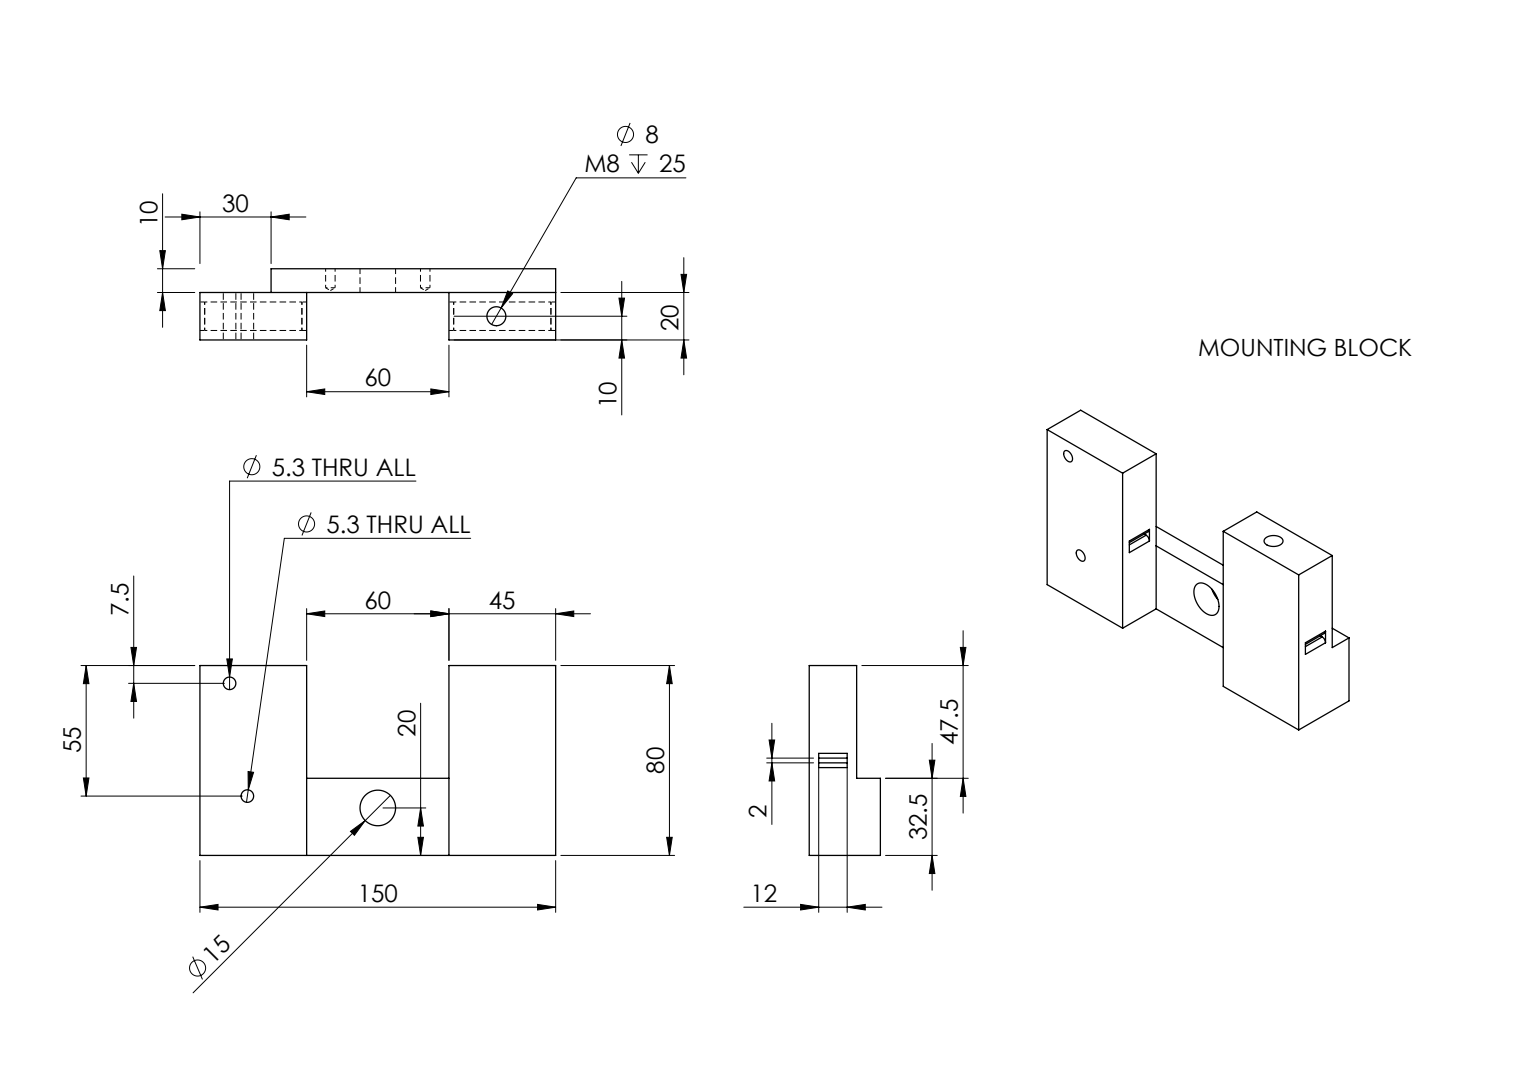
ISO-10303-21;
HEADER;
FILE_DESCRIPTION (('STEP AP214'),
    '1' );
FILE_NAME ('Mounting block.step',
    '2026-10-31T03:44:21',
    ( '' ),
    ( '' ),
    'SwSTEP 2.0',
    'SolidWorks 2026',
    '' );
FILE_SCHEMA (( 'AUTOMOTIVE_DESIGN' ));
ENDSEC;

DATA;
#10=VECTOR ( 'NONE', #15032, 1000.000000000000000 ) ;
#26=CIRCLE ( 'NONE', #5977, 1.999999999999998224 ) ;
#31=DIRECTION ( 'NONE',  ( -0.000000000000000000, 1.000000000000000000, -0.000000000000000000 ) ) ;
#35=DIRECTION ( 'NONE',  ( -1.000000000000000000, 0.000000000000000000, 0.000000000000000000 ) ) ;
#45=ORIENTED_EDGE ( 'NONE', *, *, #3522, .F. ) ;
#50=EDGE_CURVE ( 'NONE', #8587, #13131, #8250, .T. ) ;
#54=VECTOR ( 'NONE', #3678, 1000.000000000000000 ) ;
#66=DIRECTION ( 'NONE',  ( -1.000000000000000000, 0.000000000000000000, 0.000000000000000000 ) ) ;
#98=EDGE_LOOP ( 'NONE', ( #16825, #4410, #16982, #5745 ) ) ;
#99=DIRECTION ( 'NONE',  ( -1.000000000000000000, 0.000000000000000000, -0.000000000000000000 ) ) ;
#101=CARTESIAN_POINT ( 'NONE',  ( -74.99999999999997158, 1.000000000000000000, -5.999999999999998224 ) ) ;
#107=FACE_OUTER_BOUND ( 'NONE', #1049, .T. ) ;
#122=DIRECTION ( 'NONE',  ( -1.000000000000000000, 0.000000000000000000, 0.000000000000000000 ) ) ;
#140=LINE ( 'NONE', #4756, #15155 ) ;
#151=ORIENTED_EDGE ( 'NONE', *, *, #16122, .F. ) ;
#168=EDGE_CURVE ( 'NONE', #12513, #18552, #6292, .T. ) ;
#192=ADVANCED_FACE ( 'NONE', ( #13732 ), #15592, .F. ) ;
#220=DIRECTION ( 'NONE',  ( 0.000000000000000000, 0.000000000000000000, -1.000000000000000000 ) ) ;
#224=ADVANCED_FACE ( 'NONE', ( #6567 ), #9413, .T. ) ;
#265=EDGE_CURVE ( 'NONE', #12240, #6347, #18266, .T. ) ;
#268=ORIENTED_EDGE ( 'NONE', *, *, #16061, .T. ) ;
#269=AXIS2_PLACEMENT_3D ( 'NONE', #14296, #874, #6847 ) ;
#282=ORIENTED_EDGE ( 'NONE', *, *, #2242, .F. ) ;
#289=DIRECTION ( 'NONE',  ( -0.000000000000000000, -0.000000000000000000, -1.000000000000000000 ) ) ;
#305=AXIS2_PLACEMENT_3D ( 'NONE', #18598, #17407, #12786 ) ;
#315=DIRECTION ( 'NONE',  ( -1.000000000000000000, 0.000000000000000000, 0.000000000000000000 ) ) ;
#320=EDGE_CURVE ( 'NONE', #4165, #8587, #2277, .T. ) ;
#335=CIRCLE ( 'NONE', #6899, 4.000000000000003553 ) ;
#339=DIRECTION ( 'NONE',  ( 1.000000000000000000, -0.000000000000000000, -0.000000000000000000 ) ) ;
#358=ORIENTED_EDGE ( 'NONE', *, *, #8483, .F. ) ;
#359=DIRECTION ( 'NONE',  ( -0.000000000000000000, 1.000000000000000000, -0.000000000000000000 ) ) ;
#390=CYLINDRICAL_SURFACE ( 'NONE', #7746, 1.999999999999998224 ) ;
#393=DIRECTION ( 'NONE',  ( -0.000000000000000000, -0.000000000000000000, -1.000000000000000000 ) ) ;
#400=ORIENTED_EDGE ( 'NONE', *, *, #7836, .F. ) ;
#411=ADVANCED_FACE ( 'NONE', ( #6668, #2372, #8326 ), #18944, .F. ) ;
#412=CARTESIAN_POINT ( 'NONE',  ( -54.99999999999996447, -14.99999999999998579, -10.00000000000000178 ) ) ;
#422=EDGE_CURVE ( 'NONE', #7933, #6445, #10544, .T. ) ;
#441=CARTESIAN_POINT ( 'NONE',  ( 75.00000000000000000, 40.00000000000000000, 10.00000000000000000 ) ) ;
#491=ORIENTED_EDGE ( 'NONE', *, *, #3042, .F. ) ;
#492=CARTESIAN_POINT ( 'NONE',  ( 30.00000000000000000, -3.000000000000000000, 6.000000000000003553 ) ) ;
#514=VERTEX_POINT ( 'NONE', #4873 ) ;
#528=ORIENTED_EDGE ( 'NONE', *, *, #3643, .F. ) ;
#532=VECTOR ( 'NONE', #14870, 1000.000000000000000 ) ;
#535=CARTESIAN_POINT ( 'NONE',  ( -74.99999999999997158, 40.00000000000001421, -10.00000000000000000 ) ) ;
#559=CARTESIAN_POINT ( 'NONE',  ( -72.99999999999997158, 1.000000000000000000, 6.000000000000000000 ) ) ;
#562=DIRECTION ( 'NONE',  ( -1.000000000000000000, 0.000000000000000000, 0.000000000000000000 ) ) ;
#590=VERTEX_POINT ( 'NONE', #18317 ) ;
#613=ORIENTED_EDGE ( 'NONE', *, *, #8437, .T. ) ;
#619=AXIS2_PLACEMENT_3D ( 'NONE', #15609, #14025, #15907 ) ;
#628=VERTEX_POINT ( 'NONE', #2031 ) ;
#662=AXIS2_PLACEMENT_3D ( 'NONE', #14086, #13891, #15467 ) ;
#685=ORIENTED_EDGE ( 'NONE', *, *, #11171, .T. ) ;
#689=ORIENTED_EDGE ( 'NONE', *, *, #14219, .T. ) ;
#690=CARTESIAN_POINT ( 'NONE',  ( -29.99999999999999645, 40.00000000000000000, -9.999999999999998224 ) ) ;
#693=ORIENTED_EDGE ( 'NONE', *, *, #17667, .F. ) ;
#694=LINE ( 'NONE', #6666, #10977 ) ;
#706=( NAMED_UNIT ( * ) PLANE_ANGLE_UNIT ( ) SI_UNIT ( $, .RADIAN. ) );
#707=ADVANCED_FACE ( 'NONE', ( #9553 ), #15544, .F. ) ;
#710=EDGE_CURVE ( 'NONE', #5344, #15631, #17127, .T. ) ;
#714=LINE ( 'NONE', #15224, #7109 ) ;
#717=LINE ( 'NONE', #6688, #13278 ) ;
#725=CYLINDRICAL_SURFACE ( 'NONE', #9088, 1.999999999999998224 ) ;
#737=VERTEX_POINT ( 'NONE', #15940 ) ;
#752=EDGE_CURVE ( 'NONE', #928, #17028, #8377, .T. ) ;
#757=ORIENTED_EDGE ( 'NONE', *, *, #3293, .T. ) ;
#784=CARTESIAN_POINT ( 'NONE',  ( -52.34999999999998010, -14.99999999999998579, 10.00000000000000000 ) ) ;
#793=LINE ( 'NONE', #14596, #4213 ) ;
#810=CARTESIAN_POINT ( 'NONE',  ( -74.99999999999997158, -3.000000000000000000, -20.00000000000000000 ) ) ;
#829=CARTESIAN_POINT ( 'NONE',  ( -32.00000000000000000, 3.000000000000000000, 5.999999999999998224 ) ) ;
#862=CARTESIAN_POINT ( 'NONE',  ( -74.99999999999997158, -1.000000000000000000, 6.000000000000001776 ) ) ;
#868=AXIS2_PLACEMENT_3D ( 'NONE', #16000, #8438, #3843 ) ;
#872=VECTOR ( 'NONE', #8868, 1000.000000000000000 ) ;
#874=DIRECTION ( 'NONE',  ( 0.000000000000000000, 0.000000000000000000, -1.000000000000000000 ) ) ;
#877=EDGE_LOOP ( 'NONE', ( #6023, #12373, #14389 ) ) ;
#885=LINE ( 'NONE', #19147, #6712 ) ;
#886=EDGE_CURVE ( 'NONE', #11065, #15857, #4172, .T. ) ;
#927=DIRECTION ( 'NONE',  ( -0.000000000000000000, -0.000000000000000000, -1.000000000000000000 ) ) ;
#928=VERTEX_POINT ( 'NONE', #1810 ) ;
#942=DIRECTION ( 'NONE',  ( 0.000000000000000000, 8.673617379884036458E-16, 1.000000000000000000 ) ) ;
#949=VECTOR ( 'NONE', #14949, 1000.000000000000000 ) ;
#955=CYLINDRICAL_SURFACE ( 'NONE', #18451, 2.649999999999985700 ) ;
#961=ORIENTED_EDGE ( 'NONE', *, *, #7036, .F. ) ;
#965=VERTEX_POINT ( 'NONE', #13662 ) ;
#977=DIRECTION ( 'NONE',  ( -1.000000000000000000, 0.000000000000000000, 0.000000000000000000 ) ) ;
#987=CARTESIAN_POINT ( 'NONE',  ( -44.99999999999997158, -40.00000000000000000, -20.00000000000000000 ) ) ;
#990=AXIS2_PLACEMENT_3D ( 'NONE', #4540, #31, #11978 ) ;
#1049=EDGE_LOOP ( 'NONE', ( #15031, #13226, #13310, #15158 ) ) ;
#1058=ORIENTED_EDGE ( 'NONE', *, *, #752, .T. ) ;
#1060=ORIENTED_EDGE ( 'NONE', *, *, #4146, .T. ) ;
#1066=CARTESIAN_POINT ( 'NONE',  ( -20.00000000000000000, -19.99999999999999289, -12.00000000000000000 ) ) ;
#1070=AXIS2_PLACEMENT_3D ( 'NONE', #13183, #15838, #2422 ) ;
#1097=AXIS2_PLACEMENT_3D ( 'NONE', #2260, #17352, #14186 ) ;
#1122=VERTEX_POINT ( 'NONE', #9622 ) ;
#1123=CARTESIAN_POINT ( 'NONE',  ( 73.00000000000002842, -3.000000000000000000, 6.000000000000003553 ) ) ;
#1140=VERTEX_POINT ( 'NONE', #8159 ) ;
#1167=VERTEX_POINT ( 'NONE', #8253 ) ;
#1172=ORIENTED_EDGE ( 'NONE', *, *, #4024, .F. ) ;
#1174=DIRECTION ( 'NONE',  ( -0.000000000000000000, -0.000000000000000000, 1.000000000000000000 ) ) ;
#1188=DIRECTION ( 'NONE',  ( -0.000000000000000000, 1.000000000000000000, -0.000000000000000000 ) ) ;
#1214=ORIENTED_EDGE ( 'NONE', *, *, #7806, .F. ) ;
#1223=CARTESIAN_POINT ( 'NONE',  ( 32.00000000000000000, -1.000000000000000000, 6.000000000000001776 ) ) ;
#1230=CARTESIAN_POINT ( 'NONE',  ( -74.99999999999997158, -3.000000000000000000, 6.000000000000003553 ) ) ;
#1245=CIRCLE ( 'NONE', #619, 1.999999999999998224 ) ;
#1246=ORIENTED_EDGE ( 'NONE', *, *, #13234, .F. ) ;
#1250=EDGE_CURVE ( 'NONE', #1167, #2111, #10806, .T. ) ;
#1259=CARTESIAN_POINT ( 'NONE',  ( -72.99999999999997158, 1.000000000000000000, 6.000000000000000000 ) ) ;
#1267=PLANE ( 'NONE',  #8389 ) ;
#1272=DIRECTION ( 'NONE',  ( 1.000000000000000000, 0.000000000000000000, 0.000000000000000000 ) ) ;
#1274=CARTESIAN_POINT ( 'NONE',  ( 75.00000000000002842, -39.99999999999998579, 10.00000000000000000 ) ) ;
#1282=DIRECTION ( 'NONE',  ( 1.000000000000000000, 0.000000000000000000, 0.000000000000000000 ) ) ;
#1294=( GEOMETRIC_REPRESENTATION_CONTEXT ( 3 ) GLOBAL_UNCERTAINTY_ASSIGNED_CONTEXT ( ( #7918 ) ) GLOBAL_UNIT_ASSIGNED_CONTEXT ( ( #10001, #706, #6677 ) ) REPRESENTATION_CONTEXT ( 'NONE', 'WORKASPACE' ) );
#1300=ADVANCED_FACE ( 'NONE', ( #7077 ), #16017, .F. ) ;
#1302=VECTOR ( 'NONE', #12915, 1000.000000000000000 ) ;
#1314=CARTESIAN_POINT ( 'NONE',  ( 30.00000000000000000, -40.00000000000000000, 12.50000000000000000 ) ) ;
#1320=CARTESIAN_POINT ( 'NONE',  ( -74.99999999999997158, -1.000000000000000000, -5.999999999999998224 ) ) ;
#1327=EDGE_LOOP ( 'NONE', ( #17850, #7240, #8290, #4277 ) ) ;
#1343=VERTEX_POINT ( 'NONE', #9816 ) ;
#1413=DIRECTION ( 'NONE',  ( 0.000000000000000000, 0.000000000000000000, -1.000000000000000000 ) ) ;
#1432=LINE ( 'NONE', #11905, #949 ) ;
#1434=ORIENTED_EDGE ( 'NONE', *, *, #9969, .T. ) ;
#1445=ORIENTED_EDGE ( 'NONE', *, *, #5447, .F. ) ;
#1508=ORIENTED_EDGE ( 'NONE', *, *, #886, .T. ) ;
#1509=EDGE_CURVE ( 'NONE', #737, #8777, #5548, .T. ) ;
#1511=CARTESIAN_POINT ( 'NONE',  ( -74.99999999999997158, -40.00000000000000000, -10.00000000000000000 ) ) ;
#1528=ORIENTED_EDGE ( 'NONE', *, *, #18544, .T. ) ;
#1539=EDGE_CURVE ( 'NONE', #19206, #9345, #11488, .T. ) ;
#1543=ORIENTED_EDGE ( 'NONE', *, *, #11226, .F. ) ;
#1562=EDGE_CURVE ( 'NONE', #5733, #14876, #16310, .T. ) ;
#1572=DIRECTION ( 'NONE',  ( 0.000000000000000000, 0.000000000000000000, -1.000000000000000000 ) ) ;
#1599=AXIS2_PLACEMENT_3D ( 'NONE', #1314, #2979, #19182 ) ;
#1602=FACE_BOUND ( 'NONE', #7020, .T. ) ;
#1630=EDGE_CURVE ( 'NONE', #13816, #11065, #19042, .T. ) ;
#1644=DIRECTION ( 'NONE',  ( -0.000000000000000000, -0.000000000000000000, -1.000000000000000000 ) ) ;
#1663=CARTESIAN_POINT ( 'NONE',  ( 73.00000000000000000, 3.000000000000000000, 6.000000000000000000 ) ) ;
#1670=EDGE_CURVE ( 'NONE', #17840, #7933, #3375, .T. ) ;
#1673=LINE ( 'NONE', #1763, #11789 ) ;
#1710=ORIENTED_EDGE ( 'NONE', *, *, #14219, .F. ) ;
#1728=ORIENTED_EDGE ( 'NONE', *, *, #11541, .F. ) ;
#1763=CARTESIAN_POINT ( 'NONE',  ( 30.00000000000000000, 3.000000000000000000, 6.000000000000000000 ) ) ;
#1767=CARTESIAN_POINT ( 'NONE',  ( -74.99999999999997158, -39.99999999999998579, 10.00000000000000000 ) ) ;
#1773=ORIENTED_EDGE ( 'NONE', *, *, #11781, .T. ) ;
#1778=CIRCLE ( 'NONE', #15227, 2.649999999999985700 ) ;
#1781=CARTESIAN_POINT ( 'NONE',  ( 75.00000000000001421, -7.499999999999971578, -20.00000000000000000 ) ) ;
#1782=EDGE_CURVE ( 'NONE', #13131, #7980, #7122, .T. ) ;
#1784=LINE ( 'NONE', #18362, #7518 ) ;
#1786=CARTESIAN_POINT ( 'NONE',  ( -74.99999999999997158, 2.999999999999999112, 5.999999999999998224 ) ) ;
#1791=AXIS2_PLACEMENT_3D ( 'NONE', #862, #14184, #3611 ) ;
#1810=CARTESIAN_POINT ( 'NONE',  ( 50.00000000000000000, 15.00000000000000000, 4.000000000000003553 ) ) ;
#1818=EDGE_LOOP ( 'NONE', ( #3421, #16160, #16447, #11886 ) ) ;
#1851=ORIENTED_EDGE ( 'NONE', *, *, #2242, .T. ) ;
#1855=ORIENTED_EDGE ( 'NONE', *, *, #1562, .T. ) ;
#1861=CARTESIAN_POINT ( 'NONE',  ( 75.00000000000001421, -7.499999999999971578, -20.00000000000000000 ) ) ;
#1863=DIRECTION ( 'NONE',  ( 0.000000000000000000, 0.000000000000000000, 1.000000000000000000 ) ) ;
#1884=CARTESIAN_POINT ( 'NONE',  ( 7.500000000000003553, -20.00000000000000000, -20.00000000000000000 ) ) ;
#1896=ORIENTED_EDGE ( 'NONE', *, *, #7841, .F. ) ;
#1905=EDGE_LOOP ( 'NONE', ( #18790, #2116, #961, #19284, #17506, #19084, #2223, #5330, #6132, #3508 ) ) ;
#1907=DIRECTION ( 'NONE',  ( 0.000000000000000000, 1.000000000000000000, -8.673617379884036458E-16 ) ) ;
#1916=CARTESIAN_POINT ( 'NONE',  ( 50.00000000000000000, 15.00000000000000000, -4.000000000000003553 ) ) ;
#1920=VERTEX_POINT ( 'NONE', #13532 ) ;
#1921=STYLED_ITEM ( 'NONE', ( #19161 ), #9419 ) ;
#1922=EDGE_LOOP ( 'NONE', ( #15863, #11906, #16343, #18581 ) ) ;
#1931=CARTESIAN_POINT ( 'NONE',  ( -59.84999999999998721, 32.50000000000001421, 15.00000000000000000 ) ) ;
#1938=MANIFOLD_SOLID_BREP ( 'Fillet1', #12741 ) ;
#1974=CARTESIAN_POINT ( 'NONE',  ( -29.99999999999999645, 0.000000000000000000, -10.00000000000000000 ) ) ;
#1979=CARTESIAN_POINT ( 'NONE',  ( 75.00000000000001421, -7.499999999999971578, -10.00000000000000000 ) ) ;
#1981=DIRECTION ( 'NONE',  ( 0.000000000000000000, -1.000000000000000000, 8.673617379884035472E-16 ) ) ;
#2013=LINE ( 'NONE', #7788, #9049 ) ;
#2019=EDGE_CURVE ( 'NONE', #10823, #19206, #6361, .T. ) ;
#2031=CARTESIAN_POINT ( 'NONE',  ( -72.99999999999997158, -1.000000000000000000, 6.000000000000001776 ) ) ;
#2040=AXIS2_PLACEMENT_3D ( 'NONE', #6761, #14306, #8822 ) ;
#2047=EDGE_LOOP ( 'NONE', ( #613, #18279, #8119, #17452 ) ) ;
#2062=DIRECTION ( 'NONE',  ( 0.000000000000000000, 0.000000000000000000, -1.000000000000000000 ) ) ;
#2065=DIRECTION ( 'NONE',  ( 0.000000000000000000, 0.000000000000000000, -1.000000000000000000 ) ) ;
#2084=EDGE_CURVE ( 'NONE', #965, #1167, #16868, .T. ) ;
#2107=VECTOR ( 'NONE', #18285, 1000.000000000000000 ) ;
#2111=VERTEX_POINT ( 'NONE', #1767 ) ;
#2116=ORIENTED_EDGE ( 'NONE', *, *, #4651, .T. ) ;
#2125=CIRCLE ( 'NONE', #15895, 2.000000000000000000 ) ;
#2150=PLANE ( 'NONE',  #4228 ) ;
#2166=DIRECTION ( 'NONE',  ( -1.000000000000000000, 0.000000000000000000, 0.000000000000000000 ) ) ;
#2187=CARTESIAN_POINT ( 'NONE',  ( -65.14999999999996305, 32.50000000000001421, -10.00000000000000178 ) ) ;
#2207=EDGE_CURVE ( 'NONE', #6347, #9398, #2557, .T. ) ;
#2223=ORIENTED_EDGE ( 'NONE', *, *, #4224, .T. ) ;
#2227=ADVANCED_FACE ( 'NONE', ( #18633 ), #18670, .F. ) ;
#2229=CARTESIAN_POINT ( 'NONE',  ( 30.00000000000000355, 40.00000000000000000, 0.000000000000000000 ) ) ;
#2242=EDGE_CURVE ( 'NONE', #18552, #13579, #13641, .T. ) ;
#2260=CARTESIAN_POINT ( 'NONE',  ( 32.00000000000000000, 3.000000000000000000, -5.999999999999998224 ) ) ;
#2261=DIRECTION ( 'NONE',  ( 0.000000000000000000, 0.000000000000000000, 1.000000000000000000 ) ) ;
#2265=AXIS2_PLACEMENT_3D ( 'NONE', #10650, #9466, #13599 ) ;
#2277=LINE ( 'NONE', #2574, #15817 ) ;
#2306=DIRECTION ( 'NONE',  ( -0.000000000000000000, -1.000000000000000000, 8.673617379884035472E-16 ) ) ;
#2313=DIRECTION ( 'NONE',  ( 0.000000000000000000, 8.673617379884036458E-16, 1.000000000000000000 ) ) ;
#2315=DIRECTION ( 'NONE',  ( 0.000000000000000000, -1.000000000000000000, 8.673617379884035472E-16 ) ) ;
#2318=CARTESIAN_POINT ( 'NONE',  ( 75.00000000000001421, 3.000000000000000888, 5.999999999999998224 ) ) ;
#2339=VECTOR ( 'NONE', #1907, 1000.000000000000000 ) ;
#2372=FACE_OUTER_BOUND ( 'NONE', #14950, .T. ) ;
#2397=CARTESIAN_POINT ( 'NONE',  ( -74.99999999999997158, 40.00000000000001421, 10.00000000000000000 ) ) ;
#2412=ORIENTED_EDGE ( 'NONE', *, *, #5447, .T. ) ;
#2413=DIRECTION ( 'NONE',  ( 0.000000000000000000, -1.000000000000000000, 8.673617379884035472E-16 ) ) ;
#2422=DIRECTION ( 'NONE',  ( 0.000000000000000000, 0.000000000000000000, 1.000000000000000000 ) ) ;
#2444=CARTESIAN_POINT ( 'NONE',  ( -30.00000000000000000, 3.000000000000000000, -5.999999999999994671 ) ) ;
#2455=EDGE_CURVE ( 'NONE', #1140, #4430, #17290, .T. ) ;
#2458=EDGE_LOOP ( 'NONE', ( #13106, #3162, #17608 ) ) ;
#2467=VERTEX_POINT ( 'NONE', #18320 ) ;
#2470=AXIS2_PLACEMENT_3D ( 'NONE', #16873, #4991, #3619 ) ;
#2474=DIRECTION ( 'NONE',  ( -1.000000000000000000, 0.000000000000000000, 0.000000000000000000 ) ) ;
#2484=CIRCLE ( 'NONE', #9348, 1.999999999999998224 ) ;
#2489=CARTESIAN_POINT ( 'NONE',  ( -74.99999999999997158, 40.00000000000001421, 10.00000000000000000 ) ) ;
#2508=DIRECTION ( 'NONE',  ( -1.000000000000000000, 0.000000000000000000, 0.000000000000000000 ) ) ;
#2557=LINE ( 'NONE', #14187, #8631 ) ;
#2568=ORIENTED_EDGE ( 'NONE', *, *, #17667, .T. ) ;
#2574=CARTESIAN_POINT ( 'NONE',  ( -74.99999999999997158, -1.000000000000000000, 6.000000000000001776 ) ) ;
#2601=EDGE_CURVE ( 'NONE', #2467, #10823, #6887, .T. ) ;
#2607=DIRECTION ( 'NONE',  ( 0.8571673013836855759, 1.049727191973305147E-16, -0.5150380737757258576 ) ) ;
#2626=CARTESIAN_POINT ( 'NONE',  ( -57.64999999999994884, -14.99999999999998579, 15.00000000000000000 ) ) ;
#2658=EDGE_LOOP ( 'NONE', ( #13924, #14242 ) ) ;
#2661=DIRECTION ( 'NONE',  ( -0.000000000000000000, -0.000000000000000000, 1.000000000000000000 ) ) ;
#2663=EDGE_LOOP ( 'NONE', ( #1060, #3805, #8968, #3798, #151, #13906, #8954, #2568 ) ) ;
#2678=ORIENTED_EDGE ( 'NONE', *, *, #16129, .F. ) ;
#2682=VERTEX_POINT ( 'NONE', #10501 ) ;
#2698=DIRECTION ( 'NONE',  ( -0.000000000000000000, -0.000000000000000000, -1.000000000000000000 ) ) ;
#2702=ORIENTED_EDGE ( 'NONE', *, *, #5792, .T. ) ;
#2705=ADVANCED_FACE ( 'NONE', ( #1602, #10601 ), #7571, .F. ) ;
#2711=ORIENTED_EDGE ( 'NONE', *, *, #16035, .F. ) ;
#2713=VERTEX_POINT ( 'NONE', #19373 ) ;
#2715=FACE_OUTER_BOUND ( 'NONE', #15236, .T. ) ;
#2718=CARTESIAN_POINT ( 'NONE',  ( 50.00000000000000000, 15.00000000000000000, 0.000000000000000000 ) ) ;
#2735=DIRECTION ( 'NONE',  ( 0.000000000000000000, 0.000000000000000000, -1.000000000000000000 ) ) ;
#2749=ORIENTED_EDGE ( 'NONE', *, *, #16843, .F. ) ;
#2751=FACE_BOUND ( 'NONE', #7624, .T. ) ;
#2790=CARTESIAN_POINT ( 'NONE',  ( 20.00000000000000000, -20.00000000000000000, -20.00000000000000000 ) ) ;
#2807=DIRECTION ( 'NONE',  ( -0.000000000000000000, 1.000000000000000000, -0.000000000000000000 ) ) ;
#2813=ORIENTED_EDGE ( 'NONE', *, *, #14960, .F. ) ;
#2818=PLANE ( 'NONE',  #9336 ) ;
#2820=DIRECTION ( 'NONE',  ( 0.000000000000000000, 1.000000000000000000, 0.000000000000000000 ) ) ;
#2821=CARTESIAN_POINT ( 'NONE',  ( 73.00000000000002842, -3.000000000000000000, 6.000000000000001776 ) ) ;
#2829=DIRECTION ( 'NONE',  ( 0.000000000000000000, 8.673617379884036458E-16, 1.000000000000000000 ) ) ;
#2838=CIRCLE ( 'NONE', #13770, 2.649999999999985700 ) ;
#2851=FACE_OUTER_BOUND ( 'NONE', #1818, .T. ) ;
#2871=CARTESIAN_POINT ( 'NONE',  ( 0.000000000000000000, 0.000000000000000000, 0.000000000000000000 ) ) ;
#2878=AXIS2_PLACEMENT_3D ( 'NONE', #13205, #2829, #8398 ) ;
#2884=CARTESIAN_POINT ( 'NONE',  ( 75.00000000000001421, -7.499999999999971578, -20.00000000000000000 ) ) ;
#2892=VERTEX_POINT ( 'NONE', #13592 ) ;
#2899=ORIENTED_EDGE ( 'NONE', *, *, #5076, .T. ) ;
#2916=EDGE_LOOP ( 'NONE', ( #12928, #16925, #9402, #12399, #16147, #13199 ) ) ;
#2917=PLANE ( 'NONE',  #18962 ) ;
#2921=DIRECTION ( 'NONE',  ( 0.000000000000000000, 1.000000000000000000, 0.000000000000000000 ) ) ;
#2935=ORIENTED_EDGE ( 'NONE', *, *, #2601, .T. ) ;
#2941=DIRECTION ( 'NONE',  ( -0.000000000000000000, -0.000000000000000000, -1.000000000000000000 ) ) ;
#2944=EDGE_LOOP ( 'NONE', ( #268, #2702, #9574, #11135, #8690 ) ) ;
#2962=CARTESIAN_POINT ( 'NONE',  ( -74.99999999999997158, 2.999999999999999112, -20.00000000000000000 ) ) ;
#2971=CARTESIAN_POINT ( 'NONE',  ( 20.00000000000000000, -20.00000000000000000, -12.00000000000000000 ) ) ;
#2979=DIRECTION ( 'NONE',  ( -1.000000000000000000, 0.000000000000000000, 0.000000000000000000 ) ) ;
#3006=ORIENTED_EDGE ( 'NONE', *, *, #10604, .F. ) ;
#3036=ORIENTED_EDGE ( 'NONE', *, *, #16349, .F. ) ;
#3038=ORIENTED_EDGE ( 'NONE', *, *, #11713, .F. ) ;
#3040=ORIENTED_EDGE ( 'NONE', *, *, #17118, .T. ) ;
#3042=EDGE_CURVE ( 'NONE', #8991, #13296, #3589, .T. ) ;
#3043=CARTESIAN_POINT ( 'NONE',  ( -74.99999999999997158, -1.000000000000000000, -5.999999999999998224 ) ) ;
#3075=DIRECTION ( 'NONE',  ( 0.000000000000000000, 0.000000000000000000, -1.000000000000000000 ) ) ;
#3082=AXIS2_PLACEMENT_3D ( 'NONE', #2397, #8350, #14521 ) ;
#3083=DIRECTION ( 'NONE',  ( 0.000000000000000000, 0.000000000000000000, 1.000000000000000000 ) ) ;
#3085=VECTOR ( 'NONE', #17867, 1000.000000000000000 ) ;
#3093=ORIENTED_EDGE ( 'NONE', *, *, #12040, .T. ) ;
#3108=DIRECTION ( 'NONE',  ( -0.000000000000000000, -0.000000000000000000, -1.000000000000000000 ) ) ;
#3110=EDGE_CURVE ( 'NONE', #12100, #928, #7987, .T. ) ;
#3127=CARTESIAN_POINT ( 'NONE',  ( 75.00000000000001421, -2.999999999999995559, 10.00000000000000000 ) ) ;
#3150=DIRECTION ( 'NONE',  ( -0.000000000000000000, 1.000000000000000000, -0.000000000000000000 ) ) ;
#3156=AXIS2_PLACEMENT_3D ( 'NONE', #9071, #10534, #15063 ) ;
#3157=ORIENTED_EDGE ( 'NONE', *, *, #5919, .T. ) ;
#3162=ORIENTED_EDGE ( 'NONE', *, *, #18102, .T. ) ;
#3165=FACE_OUTER_BOUND ( 'NONE', #2916, .T. ) ;
#3167=DIRECTION ( 'NONE',  ( 1.000000000000000000, 0.000000000000000000, 0.000000000000000000 ) ) ;
#3177=CARTESIAN_POINT ( 'NONE',  ( -74.99999999999997158, -7.499999999999971578, -20.00000000000000000 ) ) ;
#3211=EDGE_LOOP ( 'NONE', ( #15466, #11129, #3893, #3157 ) ) ;
#3214=VERTEX_POINT ( 'NONE', #7301 ) ;
#3216=EDGE_LOOP ( 'NONE', ( #1434, #10455, #45, #10225, #9864, #15578, #757, #12437 ) ) ;
#3225=CARTESIAN_POINT ( 'NONE',  ( -74.99999999999997158, -1.000000000000000000, -5.999999999999998224 ) ) ;
#3230=LINE ( 'NONE', #11037, #3408 ) ;
#3237=ORIENTED_EDGE ( 'NONE', *, *, #16836, .F. ) ;
#3245=CARTESIAN_POINT ( 'NONE',  ( -74.99999999999997158, 40.00000000000001421, 10.00000000000000000 ) ) ;
#3258=DIRECTION ( 'NONE',  ( 1.000000000000000000, 0.000000000000000000, 0.000000000000000000 ) ) ;
#3267=VECTOR ( 'NONE', #14034, 1000.000000000000000 ) ;
#3271=CARTESIAN_POINT ( 'NONE',  ( -32.00000000000000000, 1.000000000000000000, 6.000000000000000000 ) ) ;
#3288=ADVANCED_FACE ( 'NONE', ( #2715 ), #17355, .F. ) ;
#3293=EDGE_CURVE ( 'NONE', #13672, #1920, #12983, .T. ) ;
#3311=CARTESIAN_POINT ( 'NONE',  ( -44.99999999999997158, -7.499999999999971578, -10.00000000000000000 ) ) ;
#3330=DIRECTION ( 'NONE',  ( 1.000000000000000000, -0.000000000000000000, -0.000000000000000000 ) ) ;
#3332=DIRECTION ( 'NONE',  ( -1.000000000000000000, -3.469446951953615175E-16, 0.000000000000000000 ) ) ;
#3347=CARTESIAN_POINT ( 'NONE',  ( -22.00000000000000000, -19.99999999999999289, -20.00000000000000000 ) ) ;
#3352=CARTESIAN_POINT ( 'NONE',  ( -32.00000000000000000, -3.000000000000000000, 6.000000000000001776 ) ) ;
#3353=FACE_OUTER_BOUND ( 'NONE', #13021, .T. ) ;
#3373=DIRECTION ( 'NONE',  ( -0.000000000000000000, -1.000000000000000000, -0.000000000000000000 ) ) ;
#3375=CIRCLE ( 'NONE', #14317, 2.000000000000000000 ) ;
#3382=ORIENTED_EDGE ( 'NONE', *, *, #3042, .T. ) ;
#3389=CARTESIAN_POINT ( 'NONE',  ( 75.00000000000001421, 3.000000000000002665, 10.00000000000000000 ) ) ;
#3390=CIRCLE ( 'NONE', #269, 2.000000000000001776 ) ;
#3392=AXIS2_PLACEMENT_3D ( 'NONE', #17067, #18553, #14097 ) ;
#3394=DIRECTION ( 'NONE',  ( 0.000000000000000000, 0.000000000000000000, 1.000000000000000000 ) ) ;
#3408=VECTOR ( 'NONE', #7814, 1000.000000000000000 ) ;
#3415=EDGE_CURVE ( 'NONE', #2892, #8396, #17999, .T. ) ;
#3421=ORIENTED_EDGE ( 'NONE', *, *, #18544, .F. ) ;
#3426=UNCERTAINTY_MEASURE_WITH_UNIT (LENGTH_MEASURE( 1.000000000000000082E-05 ), #5894, 'distance_accuracy_value', 'NONE');
#3446=LINE ( 'NONE', #1974, #8446 ) ;
#3454=CARTESIAN_POINT ( 'NONE',  ( 50.00000000000000000, 40.00000000000000000, -4.000000000000003553 ) ) ;
#3460=CARTESIAN_POINT ( 'NONE',  ( -18.00000000000000355, -19.99999999999999289, -20.00000000000000000 ) ) ;
#3485=VERTEX_POINT ( 'NONE', #5933 ) ;
#3508=ORIENTED_EDGE ( 'NONE', *, *, #7718, .F. ) ;
#3522=EDGE_CURVE ( 'NONE', #628, #7933, #140, .T. ) ;
#3537=EDGE_CURVE ( 'NONE', #9381, #9166, #15718, .T. ) ;
#3541=DIRECTION ( 'NONE',  ( -1.000000000000000000, 0.000000000000000000, 0.000000000000000000 ) ) ;
#3589=LINE ( 'NONE', #8185, #9203 ) ;
#3611=DIRECTION ( 'NONE',  ( 0.000000000000000000, 0.000000000000000000, -1.000000000000000000 ) ) ;
#3619=DIRECTION ( 'NONE',  ( -1.000000000000000000, 0.000000000000000000, 0.000000000000000000 ) ) ;
#3630=AXIS2_PLACEMENT_3D ( 'NONE', #4887, #11043, #6352 ) ;
#3633=LINE ( 'NONE', #9594, #16433 ) ;
#3643=EDGE_CURVE ( 'NONE', #8396, #5344, #717, .T. ) ;
#3657=VECTOR ( 'NONE', #11746, 1000.000000000000000 ) ;
#3667=CARTESIAN_POINT ( 'NONE',  ( -62.49999999999997158, 32.50000000000001421, -10.00000000000000178 ) ) ;
#3669=ORIENTED_EDGE ( 'NONE', *, *, #16761, .T. ) ;
#3678=DIRECTION ( 'NONE',  ( -0.000000000000000000, -0.000000000000000000, 1.000000000000000000 ) ) ;
#3697=FACE_OUTER_BOUND ( 'NONE', #12688, .T. ) ;
#3731=CARTESIAN_POINT ( 'NONE',  ( 0.000000000000000000, 0.000000000000000000, 10.00000000000000000 ) ) ;
#3743=AXIS2_PLACEMENT_3D ( 'NONE', #16107, #13342, #10402 ) ;
#3772=CARTESIAN_POINT ( 'NONE',  ( 2.449293598294706513E-15, -20.00000000000000000, -10.00000000000000000 ) ) ;
#3773=EDGE_LOOP ( 'NONE', ( #4351, #18109, #16076, #18032 ) ) ;
#3781=CARTESIAN_POINT ( 'NONE',  ( 32.00000000000000000, -3.000000000000000000, 6.000000000000003553 ) ) ;
#3798=ORIENTED_EDGE ( 'NONE', *, *, #16836, .T. ) ;
#3805=ORIENTED_EDGE ( 'NONE', *, *, #14960, .T. ) ;
#3830=DIRECTION ( 'NONE',  ( 0.000000000000000000, 0.000000000000000000, -1.000000000000000000 ) ) ;
#3842=AXIS2_PLACEMENT_3D ( 'NONE', #6622, #12599, #5148 ) ;
#3843=DIRECTION ( 'NONE',  ( 0.000000000000000000, -1.000000000000000000, 8.673617379884036458E-16 ) ) ;
#3863=LINE ( 'NONE', #5224, #17563 ) ;
#3867=DIRECTION ( 'NONE',  ( 1.000000000000000000, 0.000000000000000000, 0.000000000000000000 ) ) ;
#3875=ORIENTED_EDGE ( 'NONE', *, *, #13050, .F. ) ;
#3893=ORIENTED_EDGE ( 'NONE', *, *, #6521, .F. ) ;
#3930=DIRECTION ( 'NONE',  ( -0.000000000000000000, -1.000000000000000000, 8.673617379884035472E-16 ) ) ;
#3936=CARTESIAN_POINT ( 'NONE',  ( -29.99999999999999645, -40.00000000000000000, 10.00000000000000000 ) ) ;
#3944=EDGE_CURVE ( 'NONE', #13265, #15972, #12340, .T. ) ;
#3945=LINE ( 'NONE', #2489, #8122 ) ;
#3957=CARTESIAN_POINT ( 'NONE',  ( -18.00000000000000355, -19.99999999999999289, -12.00000000000000000 ) ) ;
#3970=ORIENTED_EDGE ( 'NONE', *, *, #16612, .F. ) ;
#3971=CARTESIAN_POINT ( 'NONE',  ( -30.00000000000000000, -3.000000000000000000, 6.000000000000001776 ) ) ;
#3996=AXIS2_PLACEMENT_3D ( 'NONE', #5678, #2661, #1272 ) ;
#4006=CARTESIAN_POINT ( 'NONE',  ( -30.00000000000000000, -7.500000000000005329, -10.00000000000000711 ) ) ;
#4023=VECTOR ( 'NONE', #12636, 1000.000000000000000 ) ;
#4024=EDGE_CURVE ( 'NONE', #4165, #13672, #19276, .T. ) ;
#4048=CIRCLE ( 'NONE', #14690, 2.000000000000000000 ) ;
#4056=ADVANCED_FACE ( 'NONE', ( #9219, #3353 ), #4911, .F. ) ;
#4062=CARTESIAN_POINT ( 'NONE',  ( -30.00000000000000000, 3.000000000000000000, 5.999999999999998224 ) ) ;
#4075=DIRECTION ( 'NONE',  ( 1.000000000000000000, -0.000000000000000000, -0.000000000000000000 ) ) ;
#4097=LINE ( 'NONE', #2444, #1302 ) ;
#4103=VECTOR ( 'NONE', #18373, 1000.000000000000000 ) ;
#4113=CYLINDRICAL_SURFACE ( 'NONE', #3996, 2.649999999999985700 ) ;
#4114=CARTESIAN_POINT ( 'NONE',  ( 75.00000000000001421, -7.499999999999971578, -20.00000000000000000 ) ) ;
#4137=EDGE_CURVE ( 'NONE', #6443, #16399, #12556, .T. ) ;
#4146=EDGE_CURVE ( 'NONE', #9743, #15873, #3633, .T. ) ;
#4165=VERTEX_POINT ( 'NONE', #1786 ) ;
#4172=LINE ( 'NONE', #2626, #16378 ) ;
#4173=DIRECTION ( 'NONE',  ( 0.000000000000000000, 0.000000000000000000, 1.000000000000000000 ) ) ;
#4181=ORIENTED_EDGE ( 'NONE', *, *, #1630, .T. ) ;
#4189=DIRECTION ( 'NONE',  ( -1.000000000000000000, 0.000000000000000000, 0.000000000000000000 ) ) ;
#4211=ORIENTED_EDGE ( 'NONE', *, *, #3537, .F. ) ;
#4213=VECTOR ( 'NONE', #2474, 1000.000000000000000 ) ;
#4216=( NAMED_UNIT ( * ) PLANE_ANGLE_UNIT ( ) SI_UNIT ( $, .RADIAN. ) );
#4224=EDGE_CURVE ( 'NONE', #2892, #6443, #793, .T. ) ;
#4226=AXIS2_PLACEMENT_3D ( 'NONE', #13829, #7756, #315 ) ;
#4228=AXIS2_PLACEMENT_3D ( 'NONE', #18151, #3332, #15470 ) ;
#4232=EDGE_CURVE ( 'NONE', #12513, #10379, #7026, .T. ) ;
#4258=EDGE_CURVE ( 'NONE', #16158, #13265, #885, .T. ) ;
#4273=EDGE_LOOP ( 'NONE', ( #15066, #16726, #693, #14964 ) ) ;
#4275=CARTESIAN_POINT ( 'NONE',  ( -74.99999999999997158, -1.000000000000000000, 6.000000000000001776 ) ) ;
#4276=AXIS2_PLACEMENT_3D ( 'NONE', #11383, #15910, #1282 ) ;
#4277=ORIENTED_EDGE ( 'NONE', *, *, #8716, .F. ) ;
#4281=ORIENTED_EDGE ( 'NONE', *, *, #15404, .F. ) ;
#4286=ORIENTED_EDGE ( 'NONE', *, *, #12078, .T. ) ;
#4296=ADVANCED_FACE ( 'NONE', ( #7158, #14206 ), #8327, .F. ) ;
#4312=VECTOR ( 'NONE', #17880, 1000.000000000000000 ) ;
#4329=CIRCLE ( 'NONE', #2470, 2.000000000000001776 ) ;
#4351=ORIENTED_EDGE ( 'NONE', *, *, #11908, .F. ) ;
#4401=ORIENTED_EDGE ( 'NONE', *, *, #1509, .F. ) ;
#4410=ORIENTED_EDGE ( 'NONE', *, *, #11713, .T. ) ;
#4418=CONICAL_SURFACE ( 'NONE', #16317, 1.999999999999998224, 1.029744259999999745 ) ;
#4430=VERTEX_POINT ( 'NONE', #10283 ) ;
#4432=SURFACE_STYLE_USAGE ( .BOTH. , #17970 ) ;
#4439=VECTOR ( 'NONE', #7550, 1000.000000000000000 ) ;
#4473=VECTOR ( 'NONE', #14745, 1000.000000000000000 ) ;
#4529=SURFACE_STYLE_FILL_AREA ( #16096 ) ;
#4540=CARTESIAN_POINT ( 'NONE',  ( 50.00000000000000000, 40.00000000000000000, 0.000000000000000000 ) ) ;
#4551=CARTESIAN_POINT ( 'NONE',  ( 18.00000000000000355, -20.00000000000000000, -12.00000000000000000 ) ) ;
#4576=EDGE_LOOP ( 'NONE', ( #9252, #17651 ) ) ;
#4577=CYLINDRICAL_SURFACE ( 'NONE', #3156, 2.000000000000001776 ) ;
#4600=CARTESIAN_POINT ( 'NONE',  ( 73.00000000000002842, -1.000000000000000000, 6.000000000000001776 ) ) ;
#4611=ADVANCED_FACE ( 'NONE', ( #18437, #10959 ), #2150, .F. ) ;
#4616=DIRECTION ( 'NONE',  ( 0.000000000000000000, 0.000000000000000000, 1.000000000000000000 ) ) ;
#4651=EDGE_CURVE ( 'NONE', #514, #11891, #18924, .T. ) ;
#4667=CARTESIAN_POINT ( 'NONE',  ( 7.500000000000003553, -20.00000000000000000, -10.00000000000000000 ) ) ;
#4674=DIRECTION ( 'NONE',  ( 0.000000000000000000, -0.000000000000000000, 1.000000000000000000 ) ) ;
#4684=ORIENTED_EDGE ( 'NONE', *, *, #14182, .F. ) ;
#4742=ADVANCED_FACE ( 'NONE', ( #11245 ), #15968, .F. ) ;
#4756=CARTESIAN_POINT ( 'NONE',  ( -74.99999999999997158, -1.000000000000000000, 6.000000000000001776 ) ) ;
#4770=LINE ( 'NONE', #535, #12181 ) ;
#4803=DIRECTION ( 'NONE',  ( 1.000000000000000000, 0.000000000000000000, 0.000000000000000000 ) ) ;
#4827=EDGE_CURVE ( 'NONE', #17914, #8147, #9227, .T. ) ;
#4866=VERTEX_POINT ( 'NONE', #8801 ) ;
#4873=CARTESIAN_POINT ( 'NONE',  ( -44.99999999999997158, -40.00000000000000000, -10.00000000000000000 ) ) ;
#4887=CARTESIAN_POINT ( 'NONE',  ( -72.99999999999997158, 2.999999999999999112, -20.00000000000000000 ) ) ;
#4888=VECTOR ( 'NONE', #4898, 1000.000000000000000 ) ;
#4894=FACE_OUTER_BOUND ( 'NONE', #7689, .T. ) ;
#4898=DIRECTION ( 'NONE',  ( -1.000000000000000000, 9.251858538542972814E-17, -0.000000000000000000 ) ) ;
#4911=PLANE ( 'NONE',  #10154 ) ;
#4938=LINE ( 'NONE', #15335, #18840 ) ;
#4991=DIRECTION ( 'NONE',  ( 0.000000000000000000, 0.000000000000000000, -1.000000000000000000 ) ) ;
#4998=VECTOR ( 'NONE', #18868, 1000.000000000000000 ) ;
#5005=AXIS2_PLACEMENT_3D ( 'NONE', #16542, #2921, #19413 ) ;
#5021=LINE ( 'NONE', #13746, #13764 ) ;
#5026=CIRCLE ( 'NONE', #17252, 1.999999999999998224 ) ;
#5041=VECTOR ( 'NONE', #12477, 999.9999999999998863 ) ;
#5045=ORIENTED_EDGE ( 'NONE', *, *, #15751, .T. ) ;
#5066=DIRECTION ( 'NONE',  ( 1.000000000000000000, 0.000000000000000000, 0.000000000000000000 ) ) ;
#5074=CARTESIAN_POINT ( 'NONE',  ( -30.00000000000000000, -40.00000000000000711, 6.000000000000035527 ) ) ;
#5076=EDGE_CURVE ( 'NONE', #16750, #3485, #5125, .T. ) ;
#5100=CARTESIAN_POINT ( 'NONE',  ( -62.49999999999997158, 32.50000000000001421, -10.00000000000000178 ) ) ;
#5121=CARTESIAN_POINT ( 'NONE',  ( 30.00000000000000000, -40.00000000000000711, 6.000000000000035527 ) ) ;
#5125=LINE ( 'NONE', #3127, #3267 ) ;
#5127=EDGE_CURVE ( 'NONE', #590, #8683, #9440, .T. ) ;
#5134=ORIENTED_EDGE ( 'NONE', *, *, #17618, .T. ) ;
#5148=DIRECTION ( 'NONE',  ( 0.000000000000000000, -1.000000000000000000, 8.673617379884036458E-16 ) ) ;
#5173=DIRECTION ( 'NONE',  ( -0.000000000000000000, -0.000000000000000000, -1.000000000000000000 ) ) ;
#5189=DIRECTION ( 'NONE',  ( -0.000000000000000000, -0.000000000000000000, -1.000000000000000000 ) ) ;
#5194=DIRECTION ( 'NONE',  ( 0.000000000000000000, 1.000000000000000000, 0.000000000000000000 ) ) ;
#5224=CARTESIAN_POINT ( 'NONE',  ( 75.00000000000002842, -1.000000000000000000, 6.000000000000001776 ) ) ;
#5233=ORIENTED_EDGE ( 'NONE', *, *, #12425, .T. ) ;
#5259=EDGE_CURVE ( 'NONE', #4866, #16750, #15782, .T. ) ;
#5305=DIRECTION ( 'NONE',  ( -0.8571673013836855759, 0.000000000000000000, -0.5150380737757258576 ) ) ;
#5330=ORIENTED_EDGE ( 'NONE', *, *, #4137, .T. ) ;
#5334=DIRECTION ( 'NONE',  ( 0.000000000000000000, 0.000000000000000000, 1.000000000000000000 ) ) ;
#5344=VERTEX_POINT ( 'NONE', #12074 ) ;
#5351=VECTOR ( 'NONE', #10747, 1000.000000000000000 ) ;
#5372=DIRECTION ( 'NONE',  ( 1.000000000000000000, 0.000000000000000000, 0.000000000000000000 ) ) ;
#5385=PLANE ( 'NONE',  #5872 ) ;
#5391=DIRECTION ( 'NONE',  ( 0.000000000000000000, 0.000000000000000000, -1.000000000000000000 ) ) ;
#5399=VECTOR ( 'NONE', #8579, 1000.000000000000000 ) ;
#5409=DIRECTION ( 'NONE',  ( -0.000000000000000000, 1.000000000000000000, -0.000000000000000000 ) ) ;
#5424=CARTESIAN_POINT ( 'NONE',  ( 75.00000000000000000, 40.00000000000000000, 10.00000000000000000 ) ) ;
#5431=ORIENTED_EDGE ( 'NONE', *, *, #168, .T. ) ;
#5447=EDGE_CURVE ( 'NONE', #17028, #15978, #14122, .T. ) ;
#5461=VERTEX_POINT ( 'NONE', #17779 ) ;
#5481=ORIENTED_EDGE ( 'NONE', *, *, #13828, .T. ) ;
#5489=CARTESIAN_POINT ( 'NONE',  ( -72.99999999999997158, -3.000000000000000000, -5.999999999999998224 ) ) ;
#5498=ORIENTED_EDGE ( 'NONE', *, *, #7764, .T. ) ;
#5529=CARTESIAN_POINT ( 'NONE',  ( -74.99999999999997158, 1.000000000000000000, 6.000000000000000000 ) ) ;
#5548=CIRCLE ( 'NONE', #12126, 2.000000000000001776 ) ;
#5562=CARTESIAN_POINT ( 'NONE',  ( 20.00000000000000000, -20.00000000000000000, -12.00000000000000000 ) ) ;
#5564=DIRECTION ( 'NONE',  ( 0.000000000000000000, 0.000000000000000000, -1.000000000000000000 ) ) ;
#5575=FACE_OUTER_BOUND ( 'NONE', #16050, .T. ) ;
#5619=ORIENTED_EDGE ( 'NONE', *, *, #17457, .T. ) ;
#5628=ORIENTED_EDGE ( 'NONE', *, *, #12078, .F. ) ;
#5638=AXIS2_PLACEMENT_3D ( 'NONE', #8596, #2735, #4189 ) ;
#5642=VECTOR ( 'NONE', #359, 1000.000000000000000 ) ;
#5644=ORIENTED_EDGE ( 'NONE', *, *, #7943, .T. ) ;
#5670=AXIS2_PLACEMENT_3D ( 'NONE', #3043, #1572, #99 ) ;
#5672=EDGE_LOOP ( 'NONE', ( #13995, #9582, #7291 ) ) ;
#5678=CARTESIAN_POINT ( 'NONE',  ( -54.99999999999996447, -14.99999999999998579, 15.00000000000000000 ) ) ;
#5683=EDGE_CURVE ( 'NONE', #7086, #15978, #16891, .T. ) ;
#5684=ORIENTED_EDGE ( 'NONE', *, *, #168, .F. ) ;
#5699=LINE ( 'NONE', #16392, #18485 ) ;
#5713=DIRECTION ( 'NONE',  ( 0.000000000000000000, 0.000000000000000000, -1.000000000000000000 ) ) ;
#5722=DIRECTION ( 'NONE',  ( 0.000000000000000000, 0.000000000000000000, -1.000000000000000000 ) ) ;
#5733=VERTEX_POINT ( 'NONE', #17478 ) ;
#5745=ORIENTED_EDGE ( 'NONE', *, *, #8716, .T. ) ;
#5762=LINE ( 'NONE', #11533, #532 ) ;
#5783=CARTESIAN_POINT ( 'NONE',  ( -74.99999999999997158, -39.99999999999998579, -20.00000000000000000 ) ) ;
#5784=AXIS2_PLACEMENT_3D ( 'NONE', #2971, #7659, #11975 ) ;
#5792=EDGE_CURVE ( 'NONE', #965, #16399, #6963, .T. ) ;
#5803=CARTESIAN_POINT ( 'NONE',  ( -62.49999999999997158, 32.50000000000001421, 15.00000000000000000 ) ) ;
#5834=CARTESIAN_POINT ( 'NONE',  ( -32.00000000000000000, 1.000000000000000000, -5.999999999999998224 ) ) ;
#5844=ORIENTED_EDGE ( 'NONE', *, *, #18887, .T. ) ;
#5860=CIRCLE ( 'NONE', #12736, 7.500000000000000888 ) ;
#5872=AXIS2_PLACEMENT_3D ( 'NONE', #16173, #9977, #14585 ) ;
#5894=( LENGTH_UNIT ( ) NAMED_UNIT ( * ) SI_UNIT ( .MILLI., .METRE. ) );
#5899=DIRECTION ( 'NONE',  ( -0.000000000000000000, -0.000000000000000000, 1.000000000000000000 ) ) ;
#5908=CONICAL_SURFACE ( 'NONE', #13116, 1.999999999999998224, 1.029744259999999745 ) ;
#5919=EDGE_CURVE ( 'NONE', #7980, #628, #13535, .T. ) ;
#5920=ADVANCED_FACE ( 'NONE', ( #107 ), #5995, .F. ) ;
#5929=CARTESIAN_POINT ( 'NONE',  ( 50.00000000000000000, 40.00000000000000000, 0.000000000000000000 ) ) ;
#5933=CARTESIAN_POINT ( 'NONE',  ( 75.00000000000002842, -2.999999999999999112, 6.000000000000003553 ) ) ;
#5942=AXIS2_PLACEMENT_3D ( 'NONE', #19083, #1413, #19383 ) ;
#5952=CARTESIAN_POINT ( 'NONE',  ( 75.00000000000001421, -7.499999999999971578, -20.00000000000000000 ) ) ;
#5968=FACE_OUTER_BOUND ( 'NONE', #5971, .T. ) ;
#5971=EDGE_LOOP ( 'NONE', ( #10212, #6988, #5431, #1851 ) ) ;
#5977=AXIS2_PLACEMENT_3D ( 'NONE', #13675, #1644, #13583 ) ;
#5985=LINE ( 'NONE', #1861, #17586 ) ;
#5995=CYLINDRICAL_SURFACE ( 'NONE', #17246, 4.000000000000003553 ) ;
#6023=ORIENTED_EDGE ( 'NONE', *, *, #18102, .F. ) ;
#6029=CARTESIAN_POINT ( 'NONE',  ( -72.99999999999997158, -3.000000000000000000, 6.000000000000005329 ) ) ;
#6079=CARTESIAN_POINT ( 'NONE',  ( -32.00000000000000000, -3.000000000000000000, -5.999999999999998224 ) ) ;
#6086=AXIS2_PLACEMENT_3D ( 'NONE', #8352, #10203, #17687 ) ;
#6118=DIRECTION ( 'NONE',  ( 0.000000000000000000, 8.673617379884036458E-16, 1.000000000000000000 ) ) ;
#6130=EDGE_LOOP ( 'NONE', ( #5498, #11202 ) ) ;
#6132=ORIENTED_EDGE ( 'NONE', *, *, #17016, .F. ) ;
#6155=FACE_OUTER_BOUND ( 'NONE', #7996, .T. ) ;
#6182=VECTOR ( 'NONE', #16036, 1000.000000000000000 ) ;
#6225=EDGE_LOOP ( 'NONE', ( #491, #5233, #9689, #6313 ) ) ;
#6226=EDGE_LOOP ( 'NONE', ( #14073, #17585, #6990, #18522 ) ) ;
#6235=ORIENTED_EDGE ( 'NONE', *, *, #19014, .T. ) ;
#6250=VERTEX_POINT ( 'NONE', #16073 ) ;
#6257=CIRCLE ( 'NONE', #15015, 1.999999999999998224 ) ;
#6263=CARTESIAN_POINT ( 'NONE',  ( 2.449293598294706513E-15, -20.00000000000000000, -20.00000000000000000 ) ) ;
#6275=CARTESIAN_POINT ( 'NONE',  ( 22.00000000000000000, -20.00000000000000000, -12.00000000000000000 ) ) ;
#6283=ORIENTED_EDGE ( 'NONE', *, *, #16061, .F. ) ;
#6292=LINE ( 'NONE', #1884, #14609 ) ;
#6297=( GEOMETRIC_REPRESENTATION_CONTEXT ( 3 ) GLOBAL_UNCERTAINTY_ASSIGNED_CONTEXT ( ( #3426 ) ) GLOBAL_UNIT_ASSIGNED_CONTEXT ( ( #5894, #19054, #8731 ) ) REPRESENTATION_CONTEXT ( 'NONE', 'WORKASPACE' ) );
#6304=LINE ( 'NONE', #10606, #15687 ) ;
#6313=ORIENTED_EDGE ( 'NONE', *, *, #14182, .T. ) ;
#6326=ORIENTED_EDGE ( 'NONE', *, *, #14802, .F. ) ;
#6335=DIRECTION ( 'NONE',  ( -0.000000000000000000, 1.000000000000000000, -0.000000000000000000 ) ) ;
#6347=VERTEX_POINT ( 'NONE', #4006 ) ;
#6352=DIRECTION ( 'NONE',  ( 1.000000000000000000, 0.000000000000000000, 0.000000000000000000 ) ) ;
#6361=LINE ( 'NONE', #18152, #13014 ) ;
#6375=DIRECTION ( 'NONE',  ( -1.000000000000000000, 0.000000000000000000, 0.000000000000000000 ) ) ;
#6376=CARTESIAN_POINT ( 'NONE',  ( -32.00000000000000000, -3.000000000000000000, 6.000000000000003553 ) ) ;
#6395=CARTESIAN_POINT ( 'NONE',  ( 75.00000000000002842, -39.99999999999998579, 10.00000000000000000 ) ) ;
#6407=VECTOR ( 'NONE', #5305, 1000.000000000000114 ) ;
#6421=DIRECTION ( 'NONE',  ( 0.000000000000000000, 8.673617379884036458E-16, 1.000000000000000000 ) ) ;
#6443=VERTEX_POINT ( 'NONE', #7235 ) ;
#6445=VERTEX_POINT ( 'NONE', #13406 ) ;
#6454=ADVANCED_FACE ( 'NONE', ( #5968 ), #10454, .F. ) ;
#6457=FACE_BOUND ( 'NONE', #10508, .T. ) ;
#6493=CARTESIAN_POINT ( 'NONE',  ( -74.99999999999997158, 1.000000000000000000, -5.999999999999998224 ) ) ;
#6508=CARTESIAN_POINT ( 'NONE',  ( -22.00000000000000000, -19.99999999999999289, -20.00000000000000000 ) ) ;
#6521=EDGE_CURVE ( 'NONE', #7980, #6445, #9558, .T. ) ;
#6541=VECTOR ( 'NONE', #13466, 1000.000000000000000 ) ;
#6542=AXIS2_PLACEMENT_3D ( 'NONE', #3772, #5334, #3867 ) ;
#6545=CARTESIAN_POINT ( 'NONE',  ( 30.00000000000000000, 3.000000000000000000, -5.999999999999998224 ) ) ;
#6546=SHAPE_REPRESENTATION ( 'Mounting block', ( #10359 ), #1294 ) ;
#6559=ORIENTED_EDGE ( 'NONE', *, *, #16885, .T. ) ;
#6567=FACE_OUTER_BOUND ( 'NONE', #4273, .T. ) ;
#6568=CIRCLE ( 'NONE', #8463, 2.649999999999985700 ) ;
#6611=LINE ( 'NONE', #10734, #5642 ) ;
#6617=ORIENTED_EDGE ( 'NONE', *, *, #15872, .T. ) ;
#6622=CARTESIAN_POINT ( 'NONE',  ( -74.99999999999997158, -1.000000000000000000, 6.000000000000001776 ) ) ;
#6637=DIRECTION ( 'NONE',  ( -0.000000000000000000, -0.000000000000000000, -1.000000000000000000 ) ) ;
#6666=CARTESIAN_POINT ( 'NONE',  ( 30.00000000000000355, -40.00000000000000000, 10.00000000000000000 ) ) ;
#6668=FACE_BOUND ( 'NONE', #6130, .T. ) ;
#6677=( NAMED_UNIT ( * ) SI_UNIT ( $, .STERADIAN. ) SOLID_ANGLE_UNIT ( ) );
#6681=CARTESIAN_POINT ( 'NONE',  ( 32.00000000000000000, 1.000000000000000000, 6.000000000000000000 ) ) ;
#6688=CARTESIAN_POINT ( 'NONE',  ( 30.00000000000000355, 0.000000000000000000, -10.00000000000000000 ) ) ;
#6712=VECTOR ( 'NONE', #8532, 1000.000000000000114 ) ;
#6740=CARTESIAN_POINT ( 'NONE',  ( 2.449293598294706513E-15, -20.00000000000000000, -10.00000000000000000 ) ) ;
#6761=CARTESIAN_POINT ( 'NONE',  ( -74.99999999999997158, 40.00000000000001421, 10.00000000000000000 ) ) ;
#6776=CARTESIAN_POINT ( 'NONE',  ( -22.00000000000000000, -19.99999999999999289, -12.00000000000000000 ) ) ;
#6847=DIRECTION ( 'NONE',  ( -1.000000000000000000, 0.000000000000000000, 0.000000000000000000 ) ) ;
#6849=CARTESIAN_POINT ( 'NONE',  ( -62.49999999999997158, 32.50000000000001421, 15.00000000000000000 ) ) ;
#6864=FACE_OUTER_BOUND ( 'NONE', #3216, .T. ) ;
#6887=LINE ( 'NONE', #3957, #14764 ) ;
#6899=AXIS2_PLACEMENT_3D ( 'NONE', #16212, #8943, #3083 ) ;
#6928=CARTESIAN_POINT ( 'NONE',  ( -54.99999999999996447, -14.99999999999998579, 15.00000000000000000 ) ) ;
#6939=FACE_OUTER_BOUND ( 'NONE', #2047, .T. ) ;
#6960=DIRECTION ( 'NONE',  ( 0.000000000000000000, 0.000000000000000000, 1.000000000000000000 ) ) ;
#6963=LINE ( 'NONE', #3936, #16615 ) ;
#6988=ORIENTED_EDGE ( 'NONE', *, *, #4232, .F. ) ;
#6990=ORIENTED_EDGE ( 'NONE', *, *, #3293, .F. ) ;
#6994=EDGE_CURVE ( 'NONE', #12100, #7086, #17018, .T. ) ;
#7020=EDGE_LOOP ( 'NONE', ( #14938, #9884, #13680, #12286 ) ) ;
#7026=CIRCLE ( 'NONE', #18005, 7.500000000000000888 ) ;
#7036=EDGE_CURVE ( 'NONE', #2713, #11891, #4938, .T. ) ;
#7077=FACE_OUTER_BOUND ( 'NONE', #17440, .T. ) ;
#7086=VERTEX_POINT ( 'NONE', #1916 ) ;
#7101=PRODUCT_DEFINITION_SHAPE ( 'NONE', 'NONE',  #17058 ) ;
#7103=DIRECTION ( 'NONE',  ( -0.000000000000000000, -0.000000000000000000, 1.000000000000000000 ) ) ;
#7109=VECTOR ( 'NONE', #11088, 1000.000000000000000 ) ;
#7122=CIRCLE ( 'NONE', #13067, 2.000000000000001776 ) ;
#7158=FACE_BOUND ( 'NONE', #14791, .T. ) ;
#7172=CARTESIAN_POINT ( 'NONE',  ( 20.00000000000000000, -20.00000000000000000, -12.00000000000000000 ) ) ;
#7189=PLANE ( 'NONE',  #9671 ) ;
#7192=LINE ( 'NONE', #13267, #6541 ) ;
#7231=DIRECTION ( 'NONE',  ( -0.000000000000000000, -0.000000000000000000, -1.000000000000000000 ) ) ;
#7235=CARTESIAN_POINT ( 'NONE',  ( -30.00000000000000000, -39.99999999999998579, -10.00000000000000000 ) ) ;
#7240=ORIENTED_EDGE ( 'NONE', *, *, #5076, .F. ) ;
#7242=CARTESIAN_POINT ( 'NONE',  ( 0.000000000000000000, 0.000000000000000000, -20.00000000000000000 ) ) ;
#7246=DIRECTION ( 'NONE',  ( -3.469446951953614682E-16, 1.000000000000000000, 0.000000000000000000 ) ) ;
#7250=EDGE_CURVE ( 'NONE', #14564, #9785, #15823, .T. ) ;
#7291=ORIENTED_EDGE ( 'NONE', *, *, #15404, .T. ) ;
#7301=CARTESIAN_POINT ( 'NONE',  ( -59.84999999999998721, 32.50000000000001421, -10.00000000000000178 ) ) ;
#7322=CARTESIAN_POINT ( 'NONE',  ( -74.99999999999997158, 40.00000000000001421, -10.00000000000000000 ) ) ;
#7340=CARTESIAN_POINT ( 'NONE',  ( -30.00000000000000000, -3.000000000000000000, -5.999999999999998224 ) ) ;
#7373=DIRECTION ( 'NONE',  ( 0.000000000000000000, 0.000000000000000000, -1.000000000000000000 ) ) ;
#7392=ORIENTED_EDGE ( 'NONE', *, *, #1250, .T. ) ;
#7393=CYLINDRICAL_SURFACE ( 'NONE', #9595, 4.000000000000003553 ) ;
#7424=VECTOR ( 'NONE', #16133, 1000.000000000000000 ) ;
#7433=ORIENTED_EDGE ( 'NONE', *, *, #6994, .T. ) ;
#7445=FACE_OUTER_BOUND ( 'NONE', #2663, .T. ) ;
#7485=VECTOR ( 'NONE', #927, 1000.000000000000000 ) ;
#7487=AXIS2_PLACEMENT_3D ( 'NONE', #10435, #13490, #66 ) ;
#7509=DIRECTION ( 'NONE',  ( -1.000000000000000000, 0.000000000000000000, 0.000000000000000000 ) ) ;
#7513=PLANE ( 'NONE',  #5005 ) ;
#7516=ORIENTED_EDGE ( 'NONE', *, *, #11542, .F. ) ;
#7518=VECTOR ( 'NONE', #3167, 1000.000000000000000 ) ;
#7522=DIRECTION ( 'NONE',  ( 0.000000000000000000, 0.000000000000000000, -1.000000000000000000 ) ) ;
#7526=DIRECTION ( 'NONE',  ( -0.000000000000000000, -0.000000000000000000, 1.000000000000000000 ) ) ;
#7550=DIRECTION ( 'NONE',  ( -0.000000000000000000, -0.000000000000000000, 1.000000000000000000 ) ) ;
#7571=PLANE ( 'NONE',  #17911 ) ;
#7579=VERTEX_POINT ( 'NONE', #12467 ) ;
#7606=ORIENTED_EDGE ( 'NONE', *, *, #7764, .F. ) ;
#7624=EDGE_LOOP ( 'NONE', ( #13108, #12044 ) ) ;
#7629=ORIENTED_EDGE ( 'NONE', *, *, #16761, .F. ) ;
#7631=ORIENTED_EDGE ( 'NONE', *, *, #18778, .F. ) ;
#7635=CARTESIAN_POINT ( 'NONE',  ( -32.00000000000000000, -1.000000000000000000, 6.000000000000001776 ) ) ;
#7639=VECTOR ( 'NONE', #13475, 1000.000000000000000 ) ;
#7659=DIRECTION ( 'NONE',  ( -0.000000000000000000, -0.000000000000000000, -1.000000000000000000 ) ) ;
#7667=CARTESIAN_POINT ( 'NONE',  ( -52.34999999999998010, -14.99999999999998579, 15.00000000000000000 ) ) ;
#7682=CARTESIAN_POINT ( 'NONE',  ( 73.00000000000000000, 1.000000000000000000, -5.999999999999998224 ) ) ;
#7689=EDGE_LOOP ( 'NONE', ( #15238, #15062, #17120, #11910 ) ) ;
#7711=ADVANCED_FACE ( 'NONE', ( #8911 ), #9006, .T. ) ;
#7718=EDGE_CURVE ( 'NONE', #13101, #2111, #17391, .T. ) ;
#7746=AXIS2_PLACEMENT_3D ( 'NONE', #9386, #289, #16574 ) ;
#7756=DIRECTION ( 'NONE',  ( -0.000000000000000000, -0.000000000000000000, -1.000000000000000000 ) ) ;
#7764=EDGE_CURVE ( 'NONE', #16855, #15857, #1778, .T. ) ;
#7766=LINE ( 'NONE', #7667, #11909 ) ;
#7786=ORIENTED_EDGE ( 'NONE', *, *, #7943, .F. ) ;
#7787=ORIENTED_EDGE ( 'NONE', *, *, #4827, .F. ) ;
#7788=CARTESIAN_POINT ( 'NONE',  ( -74.99999999999997158, 40.00000000000001421, 10.00000000000000000 ) ) ;
#7806=EDGE_CURVE ( 'NONE', #15978, #17028, #10546, .T. ) ;
#7811=VECTOR ( 'NONE', #5899, 1000.000000000000000 ) ;
#7814=DIRECTION ( 'NONE',  ( -0.000000000000000000, -1.000000000000000000, -0.000000000000000000 ) ) ;
#7836=EDGE_CURVE ( 'NONE', #17914, #8777, #10857, .T. ) ;
#7841=EDGE_CURVE ( 'NONE', #8147, #9166, #1673, .T. ) ;
#7856=ADVANCED_FACE ( 'NONE', ( #4894 ), #390, .F. ) ;
#7884=DIRECTION ( 'NONE',  ( -1.000000000000000000, 0.000000000000000000, 0.000000000000000000 ) ) ;
#7911=CARTESIAN_POINT ( 'NONE',  ( 20.00000000000000000, -20.00000000000000000, -12.00000000000000000 ) ) ;
#7917=FACE_OUTER_BOUND ( 'NONE', #8369, .T. ) ;
#7918=UNCERTAINTY_MEASURE_WITH_UNIT (LENGTH_MEASURE( 1.000000000000000082E-05 ), #10001, 'distance_accuracy_value', 'NONE');
#7932=DIRECTION ( 'NONE',  ( -1.000000000000000000, 0.000000000000000000, 0.000000000000000000 ) ) ;
#7933=VERTEX_POINT ( 'NONE', #7635 ) ;
#7939=UNCERTAINTY_MEASURE_WITH_UNIT (LENGTH_MEASURE( 1.000000000000000082E-05 ), #13431, 'distance_accuracy_value', 'NONE');
#7940=DIRECTION ( 'NONE',  ( 1.000000000000000000, -0.000000000000000000, -0.000000000000000000 ) ) ;
#7943=EDGE_CURVE ( 'NONE', #10379, #12513, #5860, .T. ) ;
#7980=VERTEX_POINT ( 'NONE', #8401 ) ;
#7987=LINE ( 'NONE', #13960, #14514 ) ;
#7996=EDGE_LOOP ( 'NONE', ( #4401, #3006, #18894, #4684 ) ) ;
#8033=CIRCLE ( 'NONE', #15237, 2.000000000000000000 ) ;
#8075=DIRECTION ( 'NONE',  ( -0.000000000000000000, -0.000000000000000000, -1.000000000000000000 ) ) ;
#8086=DIRECTION ( 'NONE',  ( 0.000000000000000000, -1.000000000000000000, 8.673617379884035472E-16 ) ) ;
#8119=ORIENTED_EDGE ( 'NONE', *, *, #4651, .F. ) ;
#8122=VECTOR ( 'NONE', #9521, 1000.000000000000000 ) ;
#8130=ADVANCED_FACE ( 'NONE', ( #15773 ), #12825, .F. ) ;
#8147=VERTEX_POINT ( 'NONE', #6545 ) ;
#8153=CARTESIAN_POINT ( 'NONE',  ( -30.00000000000000000, -3.000000000000002665, 6.000000000000003553 ) ) ;
#8155=DIRECTION ( 'NONE',  ( 0.000000000000000000, 1.000000000000000000, 0.000000000000000000 ) ) ;
#8159=CARTESIAN_POINT ( 'NONE',  ( 22.00000000000000000, -20.00000000000000000, -20.00000000000000000 ) ) ;
#8170=ORIENTED_EDGE ( 'NONE', *, *, #17899, .T. ) ;
#8174=CARTESIAN_POINT ( 'NONE',  ( -57.64999999999994884, -14.99999999999998579, 10.00000000000000000 ) ) ;
#8175=ORIENTED_EDGE ( 'NONE', *, *, #15633, .F. ) ;
#8185=CARTESIAN_POINT ( 'NONE',  ( -74.99999999999997158, 1.000000000000000000, 6.000000000000000000 ) ) ;
#8186=ADVANCED_FACE ( 'NONE', ( #6939 ), #12529, .F. ) ;
#8199=EDGE_CURVE ( 'NONE', #2892, #11964, #5762, .T. ) ;
#8208=EDGE_CURVE ( 'NONE', #13672, #590, #19222, .T. ) ;
#8222=CARTESIAN_POINT ( 'NONE',  ( -59.84999999999998721, 32.50000000000001421, 10.00000000000000000 ) ) ;
#8228=DIRECTION ( 'NONE',  ( 0.000000000000000000, 1.000000000000000000, 0.000000000000000000 ) ) ;
#8250=LINE ( 'NONE', #810, #10860 ) ;
#8253=CARTESIAN_POINT ( 'NONE',  ( -74.99999999999997158, 40.00000000000001421, 10.00000000000000000 ) ) ;
#8290=ORIENTED_EDGE ( 'NONE', *, *, #5259, .F. ) ;
#8301=CARTESIAN_POINT ( 'NONE',  ( 75.00000000000000000, 40.00000000000000000, -10.00000000000000000 ) ) ;
#8322=ADVANCED_FACE ( 'NONE', ( #10257 ), #10254, .F. ) ;
#8326=FACE_BOUND ( 'NONE', #2658, .T. ) ;
#8327=PLANE ( 'NONE',  #2040 ) ;
#8350=DIRECTION ( 'NONE',  ( -9.251858538542972814E-17, -1.000000000000000000, 0.000000000000000000 ) ) ;
#8352=CARTESIAN_POINT ( 'NONE',  ( 73.00000000000002842, -3.000000000000000000, -5.999999999999998224 ) ) ;
#8363=AXIS2_PLACEMENT_3D ( 'NONE', #2718, #2807, #4173 ) ;
#8369=EDGE_LOOP ( 'NONE', ( #12332, #10004, #10394, #3669 ) ) ;
#8377=LINE ( 'NONE', #11702, #5399 ) ;
#8389=AXIS2_PLACEMENT_3D ( 'NONE', #7242, #19230, #8899 ) ;
#8393=ORIENTED_EDGE ( 'NONE', *, *, #2084, .F. ) ;
#8396=VERTEX_POINT ( 'NONE', #13507 ) ;
#8398=DIRECTION ( 'NONE',  ( 0.000000000000000000, -1.000000000000000000, 8.673617379884035472E-16 ) ) ;
#8401=CARTESIAN_POINT ( 'NONE',  ( -72.99999999999997158, -1.000000000000000000, -5.999999999999998224 ) ) ;
#8406=DIRECTION ( 'NONE',  ( 0.000000000000000000, 1.000000000000000000, 0.000000000000000000 ) ) ;
#8412=CARTESIAN_POINT ( 'NONE',  ( 75.00000000000002842, -39.99999999999998579, -10.00000000000000000 ) ) ;
#8433=VECTOR ( 'NONE', #9452, 1000.000000000000000 ) ;
#8437=EDGE_CURVE ( 'NONE', #12240, #5733, #16744, .T. ) ;
#8438=DIRECTION ( 'NONE',  ( 0.000000000000000000, 8.673617379884036458E-16, 1.000000000000000000 ) ) ;
#8446=VECTOR ( 'NONE', #12260, 1000.000000000000000 ) ;
#8463=AXIS2_PLACEMENT_3D ( 'NONE', #5100, #2065, #12547 ) ;
#8478=ORIENTED_EDGE ( 'NONE', *, *, #11659, .F. ) ;
#8483=EDGE_CURVE ( 'NONE', #9166, #8991, #2125, .T. ) ;
#8502=AXIS2_PLACEMENT_3D ( 'NONE', #3781, #6421, #15348 ) ;
#8532=DIRECTION ( 'NONE',  ( 0.8571673013836855759, 1.049727191973305147E-16, -0.5150380737757258576 ) ) ;
#8543=CARTESIAN_POINT ( 'NONE',  ( 30.00000000000000000, 3.000000000000002665, 5.999999999999998224 ) ) ;
#8562=DIRECTION ( 'NONE',  ( 0.000000000000000000, 0.000000000000000000, -1.000000000000000000 ) ) ;
#8579=DIRECTION ( 'NONE',  ( -0.000000000000000000, 1.000000000000000000, -0.000000000000000000 ) ) ;
#8587=VERTEX_POINT ( 'NONE', #1230 ) ;
#8596=CARTESIAN_POINT ( 'NONE',  ( -54.99999999999996447, -14.99999999999998579, 10.00000000000000000 ) ) ;
#8609=ADVANCED_FACE ( 'NONE', ( #17710 ), #16840, .F. ) ;
#8631=VECTOR ( 'NONE', #8406, 1000.000000000000000 ) ;
#8642=ORIENTED_EDGE ( 'NONE', *, *, #17618, .F. ) ;
#8683=VERTEX_POINT ( 'NONE', #5834 ) ;
#8690=ORIENTED_EDGE ( 'NONE', *, *, #2207, .T. ) ;
#8707=FACE_BOUND ( 'NONE', #10738, .T. ) ;
#8714=ORIENTED_EDGE ( 'NONE', *, *, #7718, .T. ) ;
#8716=EDGE_CURVE ( 'NONE', #9785, #4866, #13186, .T. ) ;
#8731=( NAMED_UNIT ( * ) SI_UNIT ( $, .STERADIAN. ) SOLID_ANGLE_UNIT ( ) );
#8739=FACE_OUTER_BOUND ( 'NONE', #18556, .T. ) ;
#8757=CYLINDRICAL_SURFACE ( 'NONE', #5942, 2.000000000000001776 ) ;
#8777=VERTEX_POINT ( 'NONE', #7682 ) ;
#8783=DIRECTION ( 'NONE',  ( 1.000000000000000000, 0.000000000000000000, 0.000000000000000000 ) ) ;
#8784=DIRECTION ( 'NONE',  ( 0.000000000000000000, 0.000000000000000000, -1.000000000000000000 ) ) ;
#8799=COLOUR_RGB ( '',0.8941176470588234615, 0.8941176470588234615, 0.8941176470588234615 ) ;
#8801=CARTESIAN_POINT ( 'NONE',  ( 73.00000000000002842, -1.000000000000000000, -5.999999999999998224 ) ) ;
#8822=DIRECTION ( 'NONE',  ( 1.000000000000000000, -9.251858538542972814E-17, 0.000000000000000000 ) ) ;
#8834=DIRECTION ( 'NONE',  ( 0.000000000000000000, 0.000000000000000000, 1.000000000000000000 ) ) ;
#8868=DIRECTION ( 'NONE',  ( 0.000000000000000000, 0.000000000000000000, -1.000000000000000000 ) ) ;
#8899=DIRECTION ( 'NONE',  ( -1.000000000000000000, 0.000000000000000000, 0.000000000000000000 ) ) ;
#8906=EDGE_LOOP ( 'NONE', ( #18500, #5619, #1855, #5134 ) ) ;
#8911=FACE_OUTER_BOUND ( 'NONE', #13407, .T. ) ;
#8917=ADVANCED_FACE ( 'NONE', ( #14758 ), #2917, .F. ) ;
#8931=EDGE_CURVE ( 'NONE', #11964, #12225, #10531, .T. ) ;
#8943=DIRECTION ( 'NONE',  ( -0.000000000000000000, 1.000000000000000000, -0.000000000000000000 ) ) ;
#8954=ORIENTED_EDGE ( 'NONE', *, *, #6521, .T. ) ;
#8956=CARTESIAN_POINT ( 'NONE',  ( 30.00000000000000355, 0.000000000000000000, -10.00000000000000000 ) ) ;
#8968=ORIENTED_EDGE ( 'NONE', *, *, #5127, .F. ) ;
#8990=ORIENTED_EDGE ( 'NONE', *, *, #13409, .T. ) ;
#8991=VERTEX_POINT ( 'NONE', #6681 ) ;
#9006=CYLINDRICAL_SURFACE ( 'NONE', #4276, 2.000000000000001776 ) ;
#9020=VECTOR ( 'NONE', #19333, 1000.000000000000000 ) ;
#9025=CARTESIAN_POINT ( 'NONE',  ( 50.00000000000000000, 40.00000000000000000, 4.000000000000003553 ) ) ;
#9049=VECTOR ( 'NONE', #3108, 1000.000000000000000 ) ;
#9069=EDGE_CURVE ( 'NONE', #2467, #2682, #9710, .T. ) ;
#9071=CARTESIAN_POINT ( 'NONE',  ( 32.00000000000000000, -3.000000000000000000, 6.000000000000001776 ) ) ;
#9078=VECTOR ( 'NONE', #16062, 1000.000000000000000 ) ;
#9088=AXIS2_PLACEMENT_3D ( 'NONE', #17499, #14445, #17306 ) ;
#9112=AXIS2_PLACEMENT_3D ( 'NONE', #6079, #12624, #12333 ) ;
#9127=DIRECTION ( 'NONE',  ( 0.000000000000000000, 0.000000000000000000, -1.000000000000000000 ) ) ;
#9133=DIRECTION ( 'NONE',  ( -1.000000000000000000, 0.000000000000000000, 0.000000000000000000 ) ) ;
#9152=DIRECTION ( 'NONE',  ( 0.000000000000000000, 0.000000000000000000, 1.000000000000000000 ) ) ;
#9166=VERTEX_POINT ( 'NONE', #8543 ) ;
#9174=CARTESIAN_POINT ( 'NONE',  ( -7.499999999999998224, -20.00000000000000000, -20.00000000000000000 ) ) ;
#9177=EDGE_LOOP ( 'NONE', ( #15272, #17047, #12482 ) ) ;
#9188=ORIENTED_EDGE ( 'NONE', *, *, #3415, .T. ) ;
#9190=CARTESIAN_POINT ( 'NONE',  ( -52.34999999999998010, -14.99999999999998579, -10.00000000000000178 ) ) ;
#9203=VECTOR ( 'NONE', #12597, 1000.000000000000000 ) ;
#9219=FACE_BOUND ( 'NONE', #13463, .T. ) ;
#9227=CIRCLE ( 'NONE', #1097, 2.000000000000001776 ) ;
#9252=ORIENTED_EDGE ( 'NONE', *, *, #1630, .F. ) ;
#9266=CARTESIAN_POINT ( 'NONE',  ( -32.00000000000000000, -1.000000000000000000, -5.999999999999998224 ) ) ;
#9275=APPLICATION_CONTEXT ( 'automotive_design' ) ;
#9277=FACE_BOUND ( 'NONE', #4576, .T. ) ;
#9289=AXIS2_PLACEMENT_3D ( 'NONE', #11849, #5409, #17854 ) ;
#9325=CIRCLE ( 'NONE', #9952, 2.649999999999985700 ) ;
#9336=AXIS2_PLACEMENT_3D ( 'NONE', #4275, #19106, #10340 ) ;
#9345=VERTEX_POINT ( 'NONE', #3347 ) ;
#9347=ORIENTED_EDGE ( 'NONE', *, *, #12147, .F. ) ;
#9348=AXIS2_PLACEMENT_3D ( 'NONE', #9858, #17239, #14562 ) ;
#9364=AXIS2_PLACEMENT_3D ( 'NONE', #11153, #2062, #7932 ) ;
#9381=VERTEX_POINT ( 'NONE', #492 ) ;
#9386=CARTESIAN_POINT ( 'NONE',  ( 20.00000000000000000, -20.00000000000000000, -20.00000000000000000 ) ) ;
#9398=VERTEX_POINT ( 'NONE', #690 ) ;
#9402=ORIENTED_EDGE ( 'NONE', *, *, #16129, .T. ) ;
#9413=CYLINDRICAL_SURFACE ( 'NONE', #16131, 2.000000000000001776 ) ;
#9417=DIRECTION ( 'NONE',  ( -1.000000000000000000, 0.000000000000000000, 0.000000000000000000 ) ) ;
#9419=ADVANCED_BREP_SHAPE_REPRESENTATION ( '', ( #1938, #10359 ), #1294 ) ;
#9424=DIRECTION ( 'NONE',  ( 1.000000000000000000, -0.000000000000000000, -0.000000000000000000 ) ) ;
#9440=LINE ( 'NONE', #6493, #16104 ) ;
#9452=DIRECTION ( 'NONE',  ( -0.000000000000000000, -0.000000000000000000, -1.000000000000000000 ) ) ;
#9466=DIRECTION ( 'NONE',  ( -0.000000000000000000, -0.000000000000000000, -1.000000000000000000 ) ) ;
#9504=DIRECTION ( 'NONE',  ( 0.000000000000000000, 8.673617379884036458E-16, 1.000000000000000000 ) ) ;
#9521=DIRECTION ( 'NONE',  ( -1.000000000000000000, 9.251858538542972814E-17, -0.000000000000000000 ) ) ;
#9534=CARTESIAN_POINT ( 'NONE',  ( -74.99999999999997158, -1.000000000000000000, 6.000000000000001776 ) ) ;
#9553=FACE_OUTER_BOUND ( 'NONE', #17740, .T. ) ;
#9558=LINE ( 'NONE', #3225, #5351 ) ;
#9574=ORIENTED_EDGE ( 'NONE', *, *, #4137, .F. ) ;
#9582=ORIENTED_EDGE ( 'NONE', *, *, #9069, .T. ) ;
#9594=CARTESIAN_POINT ( 'NONE',  ( -30.00000000000000000, -40.00000000000000000, -5.999999999999998224 ) ) ;
#9595=AXIS2_PLACEMENT_3D ( 'NONE', #5929, #11890, #9152 ) ;
#9617=LINE ( 'NONE', #10714, #11476 ) ;
#9622=CARTESIAN_POINT ( 'NONE',  ( -74.99999999999997158, 2.999999999999999112, -5.999999999999998224 ) ) ;
#9671=AXIS2_PLACEMENT_3D ( 'NONE', #1320, #17607, #11882 ) ;
#9676=ADVANCED_FACE ( 'NONE', ( #2851 ), #11549, .F. ) ;
#9689=ORIENTED_EDGE ( 'NONE', *, *, #7836, .T. ) ;
#9710=LINE ( 'NONE', #6776, #6407 ) ;
#9743=VERTEX_POINT ( 'NONE', #7340 ) ;
#9775=CARTESIAN_POINT ( 'NONE',  ( -57.64999999999994884, -14.99999999999998579, -10.00000000000000178 ) ) ;
#9784=ORIENTED_EDGE ( 'NONE', *, *, #13234, .T. ) ;
#9785=VERTEX_POINT ( 'NONE', #4600 ) ;
#9816=CARTESIAN_POINT ( 'NONE',  ( 75.00000000000001421, -7.499999999999971578, -10.00000000000000000 ) ) ;
#9844=EDGE_CURVE ( 'NONE', #13265, #1140, #13609, .T. ) ;
#9858=CARTESIAN_POINT ( 'NONE',  ( -20.00000000000000000, -19.99999999999999289, -12.00000000000000000 ) ) ;
#9864=ORIENTED_EDGE ( 'NONE', *, *, #320, .F. ) ;
#9881=AXIS2_PLACEMENT_3D ( 'NONE', #1066, #5173, #17152 ) ;
#9884=ORIENTED_EDGE ( 'NONE', *, *, #320, .T. ) ;
#9933=EDGE_LOOP ( 'NONE', ( #4211, #8990, #5628, #14239 ) ) ;
#9950=ORIENTED_EDGE ( 'NONE', *, *, #14474, .T. ) ;
#9952=AXIS2_PLACEMENT_3D ( 'NONE', #19031, #11151, #977 ) ;
#9969=EDGE_CURVE ( 'NONE', #14655, #17840, #18533, .T. ) ;
#9975=ADVANCED_FACE ( 'NONE', ( #15463 ), #15274, .T. ) ;
#9977=DIRECTION ( 'NONE',  ( 0.000000000000000000, 0.000000000000000000, -1.000000000000000000 ) ) ;
#10001=( LENGTH_UNIT ( ) NAMED_UNIT ( * ) SI_UNIT ( .MILLI., .METRE. ) );
#10004=ORIENTED_EDGE ( 'NONE', *, *, #17118, .F. ) ;
#10009=LINE ( 'NONE', #11866, #7811 ) ;
#10040=CIRCLE ( 'NONE', #9112, 2.000000000000001776 ) ;
#10061=ORIENTED_EDGE ( 'NONE', *, *, #265, .F. ) ;
#10109=CARTESIAN_POINT ( 'NONE',  ( -29.99999999999999645, -40.00000000000000000, 10.00000000000000000 ) ) ;
#10127=CARTESIAN_POINT ( 'NONE',  ( 50.00000000000000000, 40.00000000000000000, -4.000000000000003553 ) ) ;
#10154=AXIS2_PLACEMENT_3D ( 'NONE', #12651, #10882, #6375 ) ;
#10175=ORIENTED_EDGE ( 'NONE', *, *, #4232, .T. ) ;
#10195=DIRECTION ( 'NONE',  ( -0.000000000000000000, -0.000000000000000000, -1.000000000000000000 ) ) ;
#10196=CYLINDRICAL_SURFACE ( 'NONE', #3743, 7.500000000000000888 ) ;
#10203=DIRECTION ( 'NONE',  ( 0.000000000000000000, 0.000000000000000000, -1.000000000000000000 ) ) ;
#10212=ORIENTED_EDGE ( 'NONE', *, *, #18036, .F. ) ;
#10218=DIRECTION ( 'NONE',  ( 1.000000000000000000, 0.000000000000000000, 0.000000000000000000 ) ) ;
#10225=ORIENTED_EDGE ( 'NONE', *, *, #11908, .T. ) ;
#10254=CONICAL_SURFACE ( 'NONE', #11809, 1.999999999999998224, 1.029744259999999745 ) ;
#10257=FACE_OUTER_BOUND ( 'NONE', #2458, .T. ) ;
#10266=CARTESIAN_POINT ( 'NONE',  ( -7.499999999999998224, -20.00000000000000000, -10.00000000000000000 ) ) ;
#10278=DIRECTION ( 'NONE',  ( -0.000000000000000000, 1.000000000000000000, -0.000000000000000000 ) ) ;
#10283=CARTESIAN_POINT ( 'NONE',  ( 18.00000000000000355, -20.00000000000000000, -20.00000000000000000 ) ) ;
#10298=CYLINDRICAL_SURFACE ( 'NONE', #11248, 2.649999999999985700 ) ;
#10311=CARTESIAN_POINT ( 'NONE',  ( -54.99999999999996447, -14.99999999999998579, -10.00000000000000178 ) ) ;
#10319=EDGE_CURVE ( 'NONE', #14876, #1343, #14959, .T. ) ;
#10340=DIRECTION ( 'NONE',  ( 0.000000000000000000, 0.000000000000000000, -1.000000000000000000 ) ) ;
#10359=AXIS2_PLACEMENT_3D ( 'NONE', #2871, #8834, #16191 ) ;
#10379=VERTEX_POINT ( 'NONE', #9174 ) ;
#10394=ORIENTED_EDGE ( 'NONE', *, *, #8931, .T. ) ;
#10395=CARTESIAN_POINT ( 'NONE',  ( -74.99999999999997158, -40.00000000000000000, -10.00000000000000000 ) ) ;
#10400=ADVANCED_FACE ( 'NONE', ( #18017 ), #4577, .T. ) ;
#10402=DIRECTION ( 'NONE',  ( 1.000000000000000000, 0.000000000000000000, 0.000000000000000000 ) ) ;
#10405=CARTESIAN_POINT ( 'NONE',  ( 73.00000000000000000, 3.000000000000000000, -5.999999999999998224 ) ) ;
#10435=CARTESIAN_POINT ( 'NONE',  ( -32.00000000000000000, 3.000000000000000000, 6.000000000000000000 ) ) ;
#10454=CYLINDRICAL_SURFACE ( 'NONE', #18207, 7.500000000000000888 ) ;
#10455=ORIENTED_EDGE ( 'NONE', *, *, #1670, .T. ) ;
#10456=EDGE_CURVE ( 'NONE', #9345, #19206, #26, .T. ) ;
#10501=CARTESIAN_POINT ( 'NONE',  ( -22.00000000000000000, -19.99999999999999289, -12.00000000000000000 ) ) ;
#10505=AXIS2_PLACEMENT_3D ( 'NONE', #6849, #1174, #11452 ) ;
#10508=EDGE_LOOP ( 'NONE', ( #14928, #1773, #14563, #11159 ) ) ;
#10519=EDGE_CURVE ( 'NONE', #514, #12240, #6611, .T. ) ;
#10531=LINE ( 'NONE', #14858, #12990 ) ;
#10534=DIRECTION ( 'NONE',  ( 0.000000000000000000, 0.000000000000000000, -1.000000000000000000 ) ) ;
#10544=LINE ( 'NONE', #9266, #16460 ) ;
#10546=CIRCLE ( 'NONE', #9289, 4.000000000000003553 ) ;
#10549=DIRECTION ( 'NONE',  ( 1.000000000000000000, 0.000000000000000000, 0.000000000000000000 ) ) ;
#10553=AXIS2_PLACEMENT_3D ( 'NONE', #412, #16889, #9417 ) ;
#10557=VECTOR ( 'NONE', #7373, 1000.000000000000000 ) ;
#10601=FACE_OUTER_BOUND ( 'NONE', #11208, .T. ) ;
#10604=EDGE_CURVE ( 'NONE', #11691, #737, #18501, .T. ) ;
#10606=CARTESIAN_POINT ( 'NONE',  ( -74.99999999999997158, -1.000000000000000000, -5.999999999999998224 ) ) ;
#10607=EDGE_LOOP ( 'NONE', ( #13413, #2935, #18639 ) ) ;
#10650=CARTESIAN_POINT ( 'NONE',  ( 20.00000000000000000, -20.00000000000000000, -20.00000000000000000 ) ) ;
#10690=AXIS2_PLACEMENT_3D ( 'NONE', #13775, #6335, #3394 ) ;
#10714=CARTESIAN_POINT ( 'NONE',  ( 75.00000000000002842, -1.000000000000000000, -5.999999999999998224 ) ) ;
#10728=ORIENTED_EDGE ( 'NONE', *, *, #19236, .F. ) ;
#10731=DIRECTION ( 'NONE',  ( -1.000000000000000000, 9.251858538542972814E-17, -0.000000000000000000 ) ) ;
#10734=CARTESIAN_POINT ( 'NONE',  ( -44.99999999999997158, -40.00000000000000000, -10.00000000000000000 ) ) ;
#10738=EDGE_LOOP ( 'NONE', ( #17524, #15585 ) ) ;
#10747=DIRECTION ( 'NONE',  ( 1.000000000000000000, -0.000000000000000000, -0.000000000000000000 ) ) ;
#10792=CARTESIAN_POINT ( 'NONE',  ( -74.99999999999997158, 40.00000000000001421, -10.00000000000000000 ) ) ;
#10801=ORIENTED_EDGE ( 'NONE', *, *, #8483, .T. ) ;
#10806=LINE ( 'NONE', #16810, #18739 ) ;
#10811=EDGE_CURVE ( 'NONE', #3485, #9785, #15052, .T. ) ;
#10823=VERTEX_POINT ( 'NONE', #11694 ) ;
#10854=AXIS2_PLACEMENT_3D ( 'NONE', #18540, #5372, #11343 ) ;
#10857=LINE ( 'NONE', #101, #13365 ) ;
#10860=VECTOR ( 'NONE', #5713, 1000.000000000000000 ) ;
#10870=EDGE_LOOP ( 'NONE', ( #12445, #16515, #3093, #17973 ) ) ;
#10882=DIRECTION ( 'NONE',  ( -0.000000000000000000, 0.000000000000000000, -1.000000000000000000 ) ) ;
#10925=ORIENTED_EDGE ( 'NONE', *, *, #15633, .T. ) ;
#10959=FACE_OUTER_BOUND ( 'NONE', #12735, .T. ) ;
#10968=ORIENTED_EDGE ( 'NONE', *, *, #2207, .F. ) ;
#10977=VECTOR ( 'NONE', #8228, 1000.000000000000000 ) ;
#10978=CARTESIAN_POINT ( 'NONE',  ( -20.00000000000000000, -19.99999999999999289, -12.00000000000000000 ) ) ;
#10991=DIRECTION ( 'NONE',  ( -0.000000000000000000, -0.000000000000000000, 1.000000000000000000 ) ) ;
#10998=CARTESIAN_POINT ( 'NONE',  ( 32.00000000000000000, 1.000000000000000000, -5.999999999999998224 ) ) ;
#10999=LINE ( 'NONE', #16711, #2107 ) ;
#11037=CARTESIAN_POINT ( 'NONE',  ( -74.99999999999997158, -39.99999999999998579, -10.00000000000000000 ) ) ;
#11043=DIRECTION ( 'NONE',  ( 0.000000000000000000, 0.000000000000000000, 1.000000000000000000 ) ) ;
#11049=PRODUCT_DEFINITION_CONTEXT ( 'detailed design', #9275, 'design' ) ;
#11065=VERTEX_POINT ( 'NONE', #9775 ) ;
#11088=DIRECTION ( 'NONE',  ( -0.000000000000000000, -0.000000000000000000, -1.000000000000000000 ) ) ;
#11098=VECTOR ( 'NONE', #5564, 1000.000000000000000 ) ;
#11117=DIRECTION ( 'NONE',  ( 0.000000000000000000, 0.5150380737757248584, 0.8571673013836862420 ) ) ;
#11129=ORIENTED_EDGE ( 'NONE', *, *, #422, .T. ) ;
#11135=ORIENTED_EDGE ( 'NONE', *, *, #16612, .T. ) ;
#11151=DIRECTION ( 'NONE',  ( 0.000000000000000000, 0.000000000000000000, -1.000000000000000000 ) ) ;
#11153=CARTESIAN_POINT ( 'NONE',  ( -62.49999999999997158, 32.50000000000001421, 10.00000000000000000 ) ) ;
#11159=ORIENTED_EDGE ( 'NONE', *, *, #11226, .T. ) ;
#11171=EDGE_CURVE ( 'NONE', #13296, #11691, #15068, .T. ) ;
#11177=ORIENTED_EDGE ( 'NONE', *, *, #8208, .F. ) ;
#11182=VECTOR ( 'NONE', #7522, 1000.000000000000000 ) ;
#11201=ORIENTED_EDGE ( 'NONE', *, *, #710, .F. ) ;
#11202=ORIENTED_EDGE ( 'NONE', *, *, #16843, .T. ) ;
#11208=EDGE_LOOP ( 'NONE', ( #5481, #8714, #12110, #689 ) ) ;
#11226=EDGE_CURVE ( 'NONE', #14655, #15873, #4097, .T. ) ;
#11245=FACE_OUTER_BOUND ( 'NONE', #16150, .T. ) ;
#11248=AXIS2_PLACEMENT_3D ( 'NONE', #5803, #11765, #16304 ) ;
#11264=DIRECTION ( 'NONE',  ( -1.000000000000000000, 0.000000000000000000, 0.000000000000000000 ) ) ;
#11277=VERTEX_POINT ( 'NONE', #7322 ) ;
#11314=EDGE_LOOP ( 'NONE', ( #10175, #5644 ) ) ;
#11332=DIRECTION ( 'NONE',  ( -1.000000000000000000, 0.000000000000000000, -0.000000000000000000 ) ) ;
#11343=DIRECTION ( 'NONE',  ( 0.000000000000000000, 0.000000000000000000, -1.000000000000000000 ) ) ;
#11362=DIRECTION ( 'NONE',  ( -1.000000000000000000, 0.000000000000000000, -0.000000000000000000 ) ) ;
#11383=CARTESIAN_POINT ( 'NONE',  ( 32.00000000000000000, 3.000000000000000000, 6.000000000000000000 ) ) ;
#11395=AXIS2_PLACEMENT_3D ( 'NONE', #13912, #9504, #14009 ) ;
#11429=DIRECTION ( 'NONE',  ( 1.000000000000000000, 0.000000000000000000, 0.000000000000000000 ) ) ;
#11442=DIRECTION ( 'NONE',  ( -1.000000000000000000, 0.000000000000000000, 0.000000000000000000 ) ) ;
#11449=CARTESIAN_POINT ( 'NONE',  ( 7.500000000000003553, -20.00000000000000000, -20.00000000000000000 ) ) ;
#11452=DIRECTION ( 'NONE',  ( 1.000000000000000000, 0.000000000000000000, 0.000000000000000000 ) ) ;
#11473=PRODUCT ( 'Mounting block', 'Mounting block', '', ( #13631 ) ) ;
#11476=VECTOR ( 'NONE', #8155, 1000.000000000000000 ) ;
#11488=CIRCLE ( 'NONE', #15901, 1.999999999999998224 ) ;
#11533=CARTESIAN_POINT ( 'NONE',  ( 30.00000000000000355, -40.00000000000000000, 0.000000000000000000 ) ) ;
#11541=EDGE_CURVE ( 'NONE', #14564, #9381, #16970, .T. ) ;
#11542=EDGE_CURVE ( 'NONE', #3214, #14841, #12594, .T. ) ;
#11546=CARTESIAN_POINT ( 'NONE',  ( 30.00000000000000000, -3.000000000000000000, -5.999999999999998224 ) ) ;
#11549=CYLINDRICAL_SURFACE ( 'NONE', #10505, 2.649999999999985700 ) ;
#11568=PLANE ( 'NONE',  #868 ) ;
#11572=ORIENTED_EDGE ( 'NONE', *, *, #15020, .T. ) ;
#11576=AXIS2_PLACEMENT_3D ( 'NONE', #16157, #3830, #2166 ) ;
#11579=VECTOR ( 'NONE', #1188, 1000.000000000000000 ) ;
#11581=VECTOR ( 'NONE', #14862, 1000.000000000000000 ) ;
#11623=FACE_OUTER_BOUND ( 'NONE', #1327, .T. ) ;
#11627=EDGE_LOOP ( 'NONE', ( #2813, #1543, #17526, #13847 ) ) ;
#11659=EDGE_CURVE ( 'NONE', #928, #7086, #14120, .T. ) ;
#11687=FACE_OUTER_BOUND ( 'NONE', #18224, .T. ) ;
#11688=ORIENTED_EDGE ( 'NONE', *, *, #19306, .F. ) ;
#11691=VERTEX_POINT ( 'NONE', #2318 ) ;
#11694=CARTESIAN_POINT ( 'NONE',  ( -18.00000000000000355, -19.99999999999999289, -12.00000000000000000 ) ) ;
#11702=CARTESIAN_POINT ( 'NONE',  ( 50.00000000000000000, 40.00000000000000000, 4.000000000000003553 ) ) ;
#11711=CARTESIAN_POINT ( 'NONE',  ( 73.00000000000000000, 1.000000000000000000, 6.000000000000000000 ) ) ;
#11713=EDGE_CURVE ( 'NONE', #7579, #14564, #12893, .T. ) ;
#11746=DIRECTION ( 'NONE',  ( -0.000000000000000000, -0.000000000000000000, 1.000000000000000000 ) ) ;
#11765=DIRECTION ( 'NONE',  ( -0.000000000000000000, -0.000000000000000000, 1.000000000000000000 ) ) ;
#11781=EDGE_CURVE ( 'NONE', #9743, #17840, #17319, .T. ) ;
#11788=FACE_OUTER_BOUND ( 'NONE', #3773, .T. ) ;
#11789=VECTOR ( 'NONE', #16965, 1000.000000000000000 ) ;
#11809=AXIS2_PLACEMENT_3D ( 'NONE', #5562, #7231, #13209 ) ;
#11828=DIRECTION ( 'NONE',  ( -0.000000000000000000, 0.000000000000000000, -1.000000000000000000 ) ) ;
#11849=CARTESIAN_POINT ( 'NONE',  ( 50.00000000000000000, 40.00000000000000000, 0.000000000000000000 ) ) ;
#11866=CARTESIAN_POINT ( 'NONE',  ( -7.499999999999998224, -20.00000000000000000, -20.00000000000000000 ) ) ;
#11872=DIRECTION ( 'NONE',  ( -0.000000000000000000, -0.000000000000000000, -1.000000000000000000 ) ) ;
#11882=DIRECTION ( 'NONE',  ( -1.000000000000000000, 0.000000000000000000, -0.000000000000000000 ) ) ;
#11886=ORIENTED_EDGE ( 'NONE', *, *, #13361, .F. ) ;
#11890=DIRECTION ( 'NONE',  ( -0.000000000000000000, 1.000000000000000000, -0.000000000000000000 ) ) ;
#11891=VERTEX_POINT ( 'NONE', #13369 ) ;
#11905=CARTESIAN_POINT ( 'NONE',  ( -65.14999999999996305, 32.50000000000001421, 15.00000000000000000 ) ) ;
#11906=ORIENTED_EDGE ( 'NONE', *, *, #2019, .T. ) ;
#11908=EDGE_CURVE ( 'NONE', #628, #8587, #8033, .T. ) ;
#11909=VECTOR ( 'NONE', #10991, 1000.000000000000000 ) ;
#11910=ORIENTED_EDGE ( 'NONE', *, *, #12040, .F. ) ;
#11918=ORIENTED_EDGE ( 'NONE', *, *, #13828, .F. ) ;
#11957=( NAMED_UNIT ( * ) SI_UNIT ( $, .STERADIAN. ) SOLID_ANGLE_UNIT ( ) );
#11964=VERTEX_POINT ( 'NONE', #14840 ) ;
#11975=DIRECTION ( 'NONE',  ( -1.000000000000000000, 0.000000000000000000, 0.000000000000000000 ) ) ;
#11978=DIRECTION ( 'NONE',  ( 0.000000000000000000, 0.000000000000000000, 1.000000000000000000 ) ) ;
#11980=DIRECTION ( 'NONE',  ( 1.000000000000000000, 0.000000000000000000, 0.000000000000000000 ) ) ;
#12008=ADVANCED_FACE ( 'NONE', ( #16327 ), #7393, .F. ) ;
#12009=CARTESIAN_POINT ( 'NONE',  ( -74.99999999999997158, 1.000000000000000000, 6.000000000000000000 ) ) ;
#12040=EDGE_CURVE ( 'NONE', #15972, #4430, #714, .T. ) ;
#12042=ORIENTED_EDGE ( 'NONE', *, *, #8199, .T. ) ;
#12044=ORIENTED_EDGE ( 'NONE', *, *, #1539, .F. ) ;
#12074=CARTESIAN_POINT ( 'NONE',  ( 30.00000000000000355, 40.00000000000000000, -9.999999999999998224 ) ) ;
#12078=EDGE_CURVE ( 'NONE', #8147, #6250, #10999, .T. ) ;
#12080=VECTOR ( 'NONE', #14177, 1000.000000000000000 ) ;
#12084=MECHANICAL_DESIGN_GEOMETRIC_PRESENTATION_REPRESENTATION('',(#15529),#15220);
#12100=VERTEX_POINT ( 'NONE', #12667 ) ;
#12101=EDGE_LOOP ( 'NONE', ( #4286, #9784, #15683, #19327, #18407, #13383, #400, #16463 ) ) ;
#12110=ORIENTED_EDGE ( 'NONE', *, *, #1250, .F. ) ;
#12126=AXIS2_PLACEMENT_3D ( 'NONE', #10405, #3075, #9133 ) ;
#12147=EDGE_CURVE ( 'NONE', #16750, #737, #9617, .T. ) ;
#12163=DIRECTION ( 'NONE',  ( 0.000000000000000000, -1.000000000000000000, -0.000000000000000000 ) ) ;
#12167=EDGE_CURVE ( 'NONE', #8683, #1920, #15325, .T. ) ;
#12181=VECTOR ( 'NONE', #10731, 1000.000000000000000 ) ;
#12225=VERTEX_POINT ( 'NONE', #6395 ) ;
#12232=FACE_OUTER_BOUND ( 'NONE', #877, .T. ) ;
#12240=VERTEX_POINT ( 'NONE', #18380 ) ;
#12256=SHAPE_DEFINITION_REPRESENTATION ( #7101, #6546 ) ;
#12260=DIRECTION ( 'NONE',  ( 0.000000000000000000, 1.000000000000000000, 0.000000000000000000 ) ) ;
#12286=ORIENTED_EDGE ( 'NONE', *, *, #16122, .T. ) ;
#12332=ORIENTED_EDGE ( 'NONE', *, *, #16349, .T. ) ;
#12333=DIRECTION ( 'NONE',  ( -1.000000000000000000, 0.000000000000000000, 0.000000000000000000 ) ) ;
#12340=CIRCLE ( 'NONE', #5784, 1.999999999999998224 ) ;
#12363=LINE ( 'NONE', #10792, #4103 ) ;
#12368=DIRECTION ( 'NONE',  ( 0.000000000000000000, 1.000000000000000000, 0.000000000000000000 ) ) ;
#12373=ORIENTED_EDGE ( 'NONE', *, *, #4258, .T. ) ;
#12387=ORIENTED_EDGE ( 'NONE', *, *, #12623, .F. ) ;
#12399=ORIENTED_EDGE ( 'NONE', *, *, #17899, .F. ) ;
#12425=EDGE_CURVE ( 'NONE', #8991, #17914, #13343, .T. ) ;
#12437=ORIENTED_EDGE ( 'NONE', *, *, #15847, .T. ) ;
#12440=ORIENTED_EDGE ( 'NONE', *, *, #18036, .T. ) ;
#12445=ORIENTED_EDGE ( 'NONE', *, *, #9844, .F. ) ;
#12467=CARTESIAN_POINT ( 'NONE',  ( 32.00000000000000000, -1.000000000000000000, -5.999999999999998224 ) ) ;
#12477=DIRECTION ( 'NONE',  ( 1.049727191973306010E-16, 0.5150380737757248584, -0.8571673013836862420 ) ) ;
#12482=ORIENTED_EDGE ( 'NONE', *, *, #11659, .T. ) ;
#12485=CARTESIAN_POINT ( 'NONE',  ( 30.00000000000000355, 40.00000000000000000, 10.00000000000000000 ) ) ;
#12502=ADVANCED_FACE ( 'NONE', ( #18841 ), #5385, .T. ) ;
#12513=VERTEX_POINT ( 'NONE', #11449 ) ;
#12514=CYLINDRICAL_SURFACE ( 'NONE', #18146, 2.000000000000001776 ) ;
#12529=PLANE ( 'NONE',  #10854 ) ;
#12547=DIRECTION ( 'NONE',  ( -1.000000000000000000, 0.000000000000000000, 0.000000000000000000 ) ) ;
#12556=LINE ( 'NONE', #18655, #15792 ) ;
#12588=PLANE ( 'NONE',  #305 ) ;
#12594=LINE ( 'NONE', #1931, #54 ) ;
#12597=DIRECTION ( 'NONE',  ( 1.000000000000000000, -0.000000000000000000, -0.000000000000000000 ) ) ;
#12599=DIRECTION ( 'NONE',  ( 0.000000000000000000, 8.673617379884036458E-16, 1.000000000000000000 ) ) ;
#12606=ADVANCED_FACE ( 'NONE', ( #5575 ), #4113, .F. ) ;
#12623=EDGE_CURVE ( 'NONE', #1343, #17671, #15877, .T. ) ;
#12624=DIRECTION ( 'NONE',  ( 0.000000000000000000, 0.000000000000000000, -1.000000000000000000 ) ) ;
#12636=DIRECTION ( 'NONE',  ( -0.000000000000000000, 0.000000000000000000, -1.000000000000000000 ) ) ;
#12642=CARTESIAN_POINT ( 'NONE',  ( 75.00000000000002842, -39.99999999999998579, 10.00000000000000000 ) ) ;
#12651=CARTESIAN_POINT ( 'NONE',  ( 0.000000000000000000, 0.000000000000000000, -10.00000000000000000 ) ) ;
#12667=CARTESIAN_POINT ( 'NONE',  ( 50.00000000000000000, 12.59655753109423237, 0.000000000000000000 ) ) ;
#12670=DIRECTION ( 'NONE',  ( 0.000000000000000000, 1.000000000000000000, 0.000000000000000000 ) ) ;
#12688=EDGE_LOOP ( 'NONE', ( #10968, #10061, #16751, #2711, #11918, #11688 ) ) ;
#12726=DIRECTION ( 'NONE',  ( 1.000000000000000000, 0.000000000000000000, 0.000000000000000000 ) ) ;
#12735=EDGE_LOOP ( 'NONE', ( #14977, #7629, #11572, #8642, #16999, #18766 ) ) ;
#12736=AXIS2_PLACEMENT_3D ( 'NONE', #6263, #1863, #4803 ) ;
#12741=CLOSED_SHELL ( 'NONE', ( #12606, #2227, #18814, #15202, #7856, #17975, #3288, #5920, #18056, #2705, #16700, #13630, #4056, #4611, #17673, #19055, #15866, #4296, #12502, #411, #13861, #1300, #13224, #6454, #12008, #8609, #9676, #192, #8322, #4742, #17181, #16958, #12864, #14060, #17656, #14551, #8130, #707, #8917, #8186, #15429, #224, #14170, #10400, #7711, #15441, #13826, #9975, #15998 ) ) ;
#12751=DIRECTION ( 'NONE',  ( -0.000000000000000000, -1.000000000000000000, -0.000000000000000000 ) ) ;
#12786=DIRECTION ( 'NONE',  ( 0.000000000000000000, -0.000000000000000000, 1.000000000000000000 ) ) ;
#12825=PLANE ( 'NONE',  #1791 ) ;
#12864=ADVANCED_FACE ( 'NONE', ( #6864 ), #11568, .F. ) ;
#12867=ORIENTED_EDGE ( 'NONE', *, *, #16885, .F. ) ;
#12893=LINE ( 'NONE', #1223, #7424 ) ;
#12915=DIRECTION ( 'NONE',  ( 0.000000000000000000, -0.000000000000000000, -1.000000000000000000 ) ) ;
#12928=ORIENTED_EDGE ( 'NONE', *, *, #8437, .F. ) ;
#12973=CARTESIAN_POINT ( 'NONE',  ( -30.00000000000000000, 3.000000000000002665, -5.999999999999998224 ) ) ;
#12983=LINE ( 'NONE', #5529, #19243 ) ;
#12990=VECTOR ( 'NONE', #8783, 1000.000000000000000 ) ;
#13014=VECTOR ( 'NONE', #393, 1000.000000000000000 ) ;
#13021=EDGE_LOOP ( 'NONE', ( #3970, #16536, #9188, #2678 ) ) ;
#13032=ORIENTED_EDGE ( 'NONE', *, *, #710, .T. ) ;
#13034=LINE ( 'NONE', #987, #15986 ) ;
#13050=EDGE_CURVE ( 'NONE', #1122, #4165, #17764, .T. ) ;
#13067=AXIS2_PLACEMENT_3D ( 'NONE', #5489, #19046, #11264 ) ;
#13094=FACE_OUTER_BOUND ( 'NONE', #3211, .T. ) ;
#13101=VERTEX_POINT ( 'NONE', #10395 ) ;
#13106=ORIENTED_EDGE ( 'NONE', *, *, #4258, .F. ) ;
#13108=ORIENTED_EDGE ( 'NONE', *, *, #10456, .F. ) ;
#13116=AXIS2_PLACEMENT_3D ( 'NONE', #7911, #6637, #562 ) ;
#13130=CIRCLE ( 'NONE', #6542, 7.500000000000000888 ) ;
#13131=VERTEX_POINT ( 'NONE', #13240 ) ;
#13183=CARTESIAN_POINT ( 'NONE',  ( 50.00000000000000000, 15.00000000000000000, 0.000000000000000000 ) ) ;
#13186=LINE ( 'NONE', #17623, #872 ) ;
#13199=ORIENTED_EDGE ( 'NONE', *, *, #1562, .F. ) ;
#13205=CARTESIAN_POINT ( 'NONE',  ( 73.00000000000000000, 3.000000000000000000, 5.999999999999998224 ) ) ;
#13209=DIRECTION ( 'NONE',  ( -1.000000000000000000, 0.000000000000000000, 0.000000000000000000 ) ) ;
#13224=ADVANCED_FACE ( 'NONE', ( #6457, #16685 ), #18446, .T. ) ;
#13226=ORIENTED_EDGE ( 'NONE', *, *, #5683, .T. ) ;
#13234=EDGE_CURVE ( 'NONE', #6250, #7579, #4329, .T. ) ;
#13240=CARTESIAN_POINT ( 'NONE',  ( -74.99999999999997158, -3.000000000000000000, -5.999999999999998224 ) ) ;
#13265=VERTEX_POINT ( 'NONE', #6275 ) ;
#13267=CARTESIAN_POINT ( 'NONE',  ( -29.99999999999999645, 40.00000000000000000, 0.000000000000000000 ) ) ;
#13278=VECTOR ( 'NONE', #12670, 1000.000000000000000 ) ;
#13296=VERTEX_POINT ( 'NONE', #18354 ) ;
#13310=ORIENTED_EDGE ( 'NONE', *, *, #7806, .T. ) ;
#13321=CARTESIAN_POINT ( 'NONE',  ( -54.99999999999996447, -14.99999999999998579, 10.00000000000000000 ) ) ;
#13342=DIRECTION ( 'NONE',  ( -0.000000000000000000, -0.000000000000000000, 1.000000000000000000 ) ) ;
#13343=LINE ( 'NONE', #19365, #10557 ) ;
#13358=ORIENTED_EDGE ( 'NONE', *, *, #19306, .T. ) ;
#13361=EDGE_CURVE ( 'NONE', #5461, #14841, #9325, .T. ) ;
#13365=VECTOR ( 'NONE', #3330, 1000.000000000000000 ) ;
#13369=CARTESIAN_POINT ( 'NONE',  ( -44.99999999999997158, -40.00000000000000000, -20.00000000000000000 ) ) ;
#13383=ORIENTED_EDGE ( 'NONE', *, *, #1509, .T. ) ;
#13384=DIRECTION ( 'NONE',  ( 0.000000000000000000, -0.000000000000000000, 1.000000000000000000 ) ) ;
#13406=CARTESIAN_POINT ( 'NONE',  ( -32.00000000000000000, -1.000000000000000000, -5.999999999999998224 ) ) ;
#13407=EDGE_LOOP ( 'NONE', ( #358, #1896, #7787, #17628 ) ) ;
#13409=EDGE_CURVE ( 'NONE', #9381, #6250, #17159, .T. ) ;
#13413=ORIENTED_EDGE ( 'NONE', *, *, #9069, .F. ) ;
#13431=( LENGTH_UNIT ( ) NAMED_UNIT ( * ) SI_UNIT ( .MILLI., .METRE. ) );
#13440=VECTOR ( 'NONE', #10218, 1000.000000000000000 ) ;
#13458=DIRECTION ( 'NONE',  ( -1.000000000000000000, 0.000000000000000000, 0.000000000000000000 ) ) ;
#13463=EDGE_LOOP ( 'NONE', ( #282, #13707 ) ) ;
#13466=DIRECTION ( 'NONE',  ( -0.000000000000000000, -0.000000000000000000, 1.000000000000000000 ) ) ;
#13475=DIRECTION ( 'NONE',  ( 0.000000000000000000, 1.000000000000000000, 0.000000000000000000 ) ) ;
#13488=CIRCLE ( 'NONE', #14414, 2.649999999999985700 ) ;
#13490=DIRECTION ( 'NONE',  ( 0.000000000000000000, 0.000000000000000000, -1.000000000000000000 ) ) ;
#13507=CARTESIAN_POINT ( 'NONE',  ( 30.00000000000000000, -7.499999999999971578, -10.00000000000000000 ) ) ;
#13515=ORIENTED_EDGE ( 'NONE', *, *, #18887, .F. ) ;
#13525=ORIENTED_EDGE ( 'NONE', *, *, #5683, .F. ) ;
#13532=CARTESIAN_POINT ( 'NONE',  ( -32.00000000000000000, 1.000000000000000000, 6.000000000000000000 ) ) ;
#13535=LINE ( 'NONE', #14998, #4439 ) ;
#13549=CARTESIAN_POINT ( 'NONE',  ( -20.00000000000000000, -19.99999999999999289, -20.00000000000000000 ) ) ;
#13556=FACE_BOUND ( 'NONE', #9933, .T. ) ;
#13579=VERTEX_POINT ( 'NONE', #10266 ) ;
#13582=ORIENTED_EDGE ( 'NONE', *, *, #19236, .T. ) ;
#13583=DIRECTION ( 'NONE',  ( -1.000000000000000000, 0.000000000000000000, 0.000000000000000000 ) ) ;
#13585=FACE_OUTER_BOUND ( 'NONE', #6226, .T. ) ;
#13592=CARTESIAN_POINT ( 'NONE',  ( 30.00000000000000355, -39.99999999999998579, -10.00000000000000178 ) ) ;
#13599=DIRECTION ( 'NONE',  ( -1.000000000000000000, 0.000000000000000000, 0.000000000000000000 ) ) ;
#13609=LINE ( 'NONE', #18141, #17105 ) ;
#13617=AXIS2_PLACEMENT_3D ( 'NONE', #3731, #5391, #11362 ) ;
#13618=AXIS2_PLACEMENT_3D ( 'NONE', #16070, #15869, #11442 ) ;
#13630=ADVANCED_FACE ( 'NONE', ( #2751, #8707, #16269, #14685 ), #1267, .T. ) ;
#13631=PRODUCT_CONTEXT ( 'NONE', #17284, 'mechanical' ) ;
#13641=CIRCLE ( 'NONE', #15513, 7.500000000000000888 ) ;
#13662=CARTESIAN_POINT ( 'NONE',  ( -29.99999999999999645, 40.00000000000000000, 10.00000000000000000 ) ) ;
#13669=VECTOR ( 'NONE', #14026, 1000.000000000000000 ) ;
#13672=VERTEX_POINT ( 'NONE', #559 ) ;
#13675=CARTESIAN_POINT ( 'NONE',  ( -20.00000000000000000, -19.99999999999999289, -20.00000000000000000 ) ) ;
#13680=ORIENTED_EDGE ( 'NONE', *, *, #50, .T. ) ;
#13707=ORIENTED_EDGE ( 'NONE', *, *, #14474, .F. ) ;
#13732=FACE_OUTER_BOUND ( 'NONE', #10870, .T. ) ;
#13746=CARTESIAN_POINT ( 'NONE',  ( -74.99999999999997158, -1.000000000000000000, -5.999999999999998224 ) ) ;
#13764=VECTOR ( 'NONE', #12368, 1000.000000000000000 ) ;
#13770=AXIS2_PLACEMENT_3D ( 'NONE', #3667, #8562, #2508 ) ;
#13775=CARTESIAN_POINT ( 'NONE',  ( 50.00000000000000000, 15.00000000000000000, 0.000000000000000000 ) ) ;
#13798=AXIS2_PLACEMENT_3D ( 'NONE', #1123, #15735, #2315 ) ;
#13816=VERTEX_POINT ( 'NONE', #9190 ) ;
#13826=ADVANCED_FACE ( 'NONE', ( #6155 ), #12514, .T. ) ;
#13828=EDGE_CURVE ( 'NONE', #11277, #13101, #3230, .T. ) ;
#13829=CARTESIAN_POINT ( 'NONE',  ( 20.00000000000000000, -20.00000000000000000, -20.00000000000000000 ) ) ;
#13847=ORIENTED_EDGE ( 'NONE', *, *, #12167, .F. ) ;
#13861=ADVANCED_FACE ( 'NONE', ( #9277, #18327, #3697 ), #14367, .T. ) ;
#13891=DIRECTION ( 'NONE',  ( 0.000000000000000000, 0.000000000000000000, -1.000000000000000000 ) ) ;
#13906=ORIENTED_EDGE ( 'NONE', *, *, #1782, .T. ) ;
#13912=CARTESIAN_POINT ( 'NONE',  ( -72.99999999999997158, 2.999999999999999112, 5.999999999999998224 ) ) ;
#13924=ORIENTED_EDGE ( 'NONE', *, *, #14802, .T. ) ;
#13960=CARTESIAN_POINT ( 'NONE',  ( 50.00000000000000000, 15.00000000000000000, 4.000000000000003553 ) ) ;
#13995=ORIENTED_EDGE ( 'NONE', *, *, #2601, .F. ) ;
#14009=DIRECTION ( 'NONE',  ( 0.000000000000000000, -1.000000000000000000, 8.673617379884035472E-16 ) ) ;
#14025=DIRECTION ( 'NONE',  ( -0.000000000000000000, -0.000000000000000000, -1.000000000000000000 ) ) ;
#14026=DIRECTION ( 'NONE',  ( -0.000000000000000000, 0.000000000000000000, 1.000000000000000000 ) ) ;
#14034=DIRECTION ( 'NONE',  ( -0.000000000000000000, -0.000000000000000000, 1.000000000000000000 ) ) ;
#14057=ORIENTED_EDGE ( 'NONE', *, *, #10604, .T. ) ;
#14060=ADVANCED_FACE ( 'NONE', ( #13094 ), #2818, .F. ) ;
#14073=ORIENTED_EDGE ( 'NONE', *, *, #5127, .T. ) ;
#14086=CARTESIAN_POINT ( 'NONE',  ( 0.000000000000000000, 0.000000000000000000, 10.00000000000000000 ) ) ;
#14097=DIRECTION ( 'NONE',  ( 0.000000000000000000, 0.000000000000000000, -1.000000000000000000 ) ) ;
#14120=CIRCLE ( 'NONE', #10690, 4.000000000000003553 ) ;
#14122=CIRCLE ( 'NONE', #990, 4.000000000000003553 ) ;
#14128=LINE ( 'NONE', #17387, #4998 ) ;
#14166=ORIENTED_EDGE ( 'NONE', *, *, #10811, .T. ) ;
#14167=PRODUCT_DEFINITION_FORMATION_WITH_SPECIFIED_SOURCE ( 'ANY', '', #11473, .NOT_KNOWN. ) ;
#14170=ADVANCED_FACE ( 'NONE', ( #14952 ), #19304, .T. ) ;
#14177=DIRECTION ( 'NONE',  ( -0.000000000000000000, -1.000000000000000000, 8.673617379884036458E-16 ) ) ;
#14182=EDGE_CURVE ( 'NONE', #8777, #13296, #14559, .T. ) ;
#14184=DIRECTION ( 'NONE',  ( 0.000000000000000000, -1.000000000000000000, -0.000000000000000000 ) ) ;
#14186=DIRECTION ( 'NONE',  ( -1.000000000000000000, 0.000000000000000000, 0.000000000000000000 ) ) ;
#14187=CARTESIAN_POINT ( 'NONE',  ( -29.99999999999999645, 0.000000000000000000, -10.00000000000000000 ) ) ;
#14199=CARTESIAN_POINT ( 'NONE',  ( 75.00000000000001421, -2.999999999999999112, -5.999999999999998224 ) ) ;
#14206=FACE_OUTER_BOUND ( 'NONE', #17295, .T. ) ;
#14219=EDGE_CURVE ( 'NONE', #1167, #11277, #2013, .T. ) ;
#14239=ORIENTED_EDGE ( 'NONE', *, *, #7841, .T. ) ;
#14242=ORIENTED_EDGE ( 'NONE', *, *, #13361, .T. ) ;
#14245=FACE_OUTER_BOUND ( 'NONE', #1905, .T. ) ;
#14264=VERTEX_POINT ( 'NONE', #441 ) ;
#14296=CARTESIAN_POINT ( 'NONE',  ( -32.00000000000000000, 3.000000000000000000, -5.999999999999998224 ) ) ;
#14306=DIRECTION ( 'NONE',  ( -9.251858538542972814E-17, -1.000000000000000000, 0.000000000000000000 ) ) ;
#14317=AXIS2_PLACEMENT_3D ( 'NONE', #6376, #18461, #1981 ) ;
#14367=PLANE ( 'NONE',  #17196 ) ;
#14371=FACE_OUTER_BOUND ( 'NONE', #16959, .T. ) ;
#14389=ORIENTED_EDGE ( 'NONE', *, *, #3944, .T. ) ;
#14398=ORIENTED_EDGE ( 'NONE', *, *, #2019, .F. ) ;
#14404=CIRCLE ( 'NONE', #5638, 2.649999999999985700 ) ;
#14405=DIRECTION ( 'NONE',  ( 1.000000000000000000, 0.000000000000000000, 0.000000000000000000 ) ) ;
#14414=AXIS2_PLACEMENT_3D ( 'NONE', #10311, #5722, #35 ) ;
#14445=DIRECTION ( 'NONE',  ( -0.000000000000000000, -0.000000000000000000, -1.000000000000000000 ) ) ;
#14474=EDGE_CURVE ( 'NONE', #13579, #18552, #13130, .T. ) ;
#14514=VECTOR ( 'NONE', #11117, 999.9999999999998863 ) ;
#14521=DIRECTION ( 'NONE',  ( 1.000000000000000000, -9.251858538542972814E-17, 0.000000000000000000 ) ) ;
#14551=ADVANCED_FACE ( 'NONE', ( #16216 ), #7189, .F. ) ;
#14559=LINE ( 'NONE', #11711, #18467 ) ;
#14562=DIRECTION ( 'NONE',  ( -1.000000000000000000, 0.000000000000000000, 0.000000000000000000 ) ) ;
#14563=ORIENTED_EDGE ( 'NONE', *, *, #9969, .F. ) ;
#14564=VERTEX_POINT ( 'NONE', #17695 ) ;
#14585=DIRECTION ( 'NONE',  ( -1.000000000000000000, 0.000000000000000000, -0.000000000000000000 ) ) ;
#14596=CARTESIAN_POINT ( 'NONE',  ( 75.00000000000001421, -39.99999999999998579, -10.00000000000000000 ) ) ;
#14609=VECTOR ( 'NONE', #16989, 1000.000000000000000 ) ;
#14655=VERTEX_POINT ( 'NONE', #4062 ) ;
#14685=FACE_OUTER_BOUND ( 'NONE', #8906, .T. ) ;
#14690=AXIS2_PLACEMENT_3D ( 'NONE', #829, #2313, #2413 ) ;
#14714=AXIS2_PLACEMENT_3D ( 'NONE', #1781, #12163, #9127 ) ;
#14745=DIRECTION ( 'NONE',  ( -0.000000000000000000, -0.000000000000000000, 1.000000000000000000 ) ) ;
#14758=FACE_OUTER_BOUND ( 'NONE', #6225, .T. ) ;
#14764=VECTOR ( 'NONE', #2607, 1000.000000000000114 ) ;
#14791=EDGE_LOOP ( 'NONE', ( #1445, #1214 ) ) ;
#14800=CARTESIAN_POINT ( 'NONE',  ( 50.00000000000000000, 40.00000000000000000, 0.000000000000000000 ) ) ;
#14802=EDGE_CURVE ( 'NONE', #14841, #5461, #17849, .T. ) ;
#14809=FILL_AREA_STYLE_COLOUR ( '', #8799 ) ;
#14828=PLANE ( 'NONE',  #1599 ) ;
#14840=CARTESIAN_POINT ( 'NONE',  ( 30.00000000000000355, -40.00000000000000000, 10.00000000000000000 ) ) ;
#14841=VERTEX_POINT ( 'NONE', #8222 ) ;
#14857=ORIENTED_EDGE ( 'NONE', *, *, #5792, .F. ) ;
#14858=CARTESIAN_POINT ( 'NONE',  ( -74.99999999999997158, -39.99999999999998579, 10.00000000000000000 ) ) ;
#14862=DIRECTION ( 'NONE',  ( -0.000000000000000000, -0.000000000000000000, 1.000000000000000000 ) ) ;
#14870=DIRECTION ( 'NONE',  ( -0.000000000000000000, -0.000000000000000000, 1.000000000000000000 ) ) ;
#14876=VERTEX_POINT ( 'NONE', #4114 ) ;
#14928=ORIENTED_EDGE ( 'NONE', *, *, #4146, .F. ) ;
#14930=ORIENTED_EDGE ( 'NONE', *, *, #886, .F. ) ;
#14937=DIRECTION ( 'NONE',  ( 0.000000000000000000, -1.000000000000000000, 8.673617379884035472E-16 ) ) ;
#14938=ORIENTED_EDGE ( 'NONE', *, *, #13050, .T. ) ;
#14949=DIRECTION ( 'NONE',  ( -0.000000000000000000, -0.000000000000000000, 1.000000000000000000 ) ) ;
#14950=EDGE_LOOP ( 'NONE', ( #14857, #15363, #7392, #17268 ) ) ;
#14952=FACE_OUTER_BOUND ( 'NONE', #11627, .T. ) ;
#14959=LINE ( 'NONE', #5952, #11581 ) ;
#14960=EDGE_CURVE ( 'NONE', #15873, #8683, #3390, .T. ) ;
#14963=EDGE_LOOP ( 'NONE', ( #1246, #15761, #1728, #3038 ) ) ;
#14964=ORIENTED_EDGE ( 'NONE', *, *, #422, .F. ) ;
#14977=ORIENTED_EDGE ( 'NONE', *, *, #15872, .F. ) ;
#14985=EDGE_LOOP ( 'NONE', ( #12867, #7631 ) ) ;
#14998=CARTESIAN_POINT ( 'NONE',  ( -72.99999999999997158, -1.000000000000000000, 6.000000000000001776 ) ) ;
#15015=AXIS2_PLACEMENT_3D ( 'NONE', #7172, #10195, #19166 ) ;
#15020=EDGE_CURVE ( 'NONE', #12225, #2713, #15088, .T. ) ;
#15031=ORIENTED_EDGE ( 'NONE', *, *, #18929, .F. ) ;
#15032=DIRECTION ( 'NONE',  ( 1.000000000000000000, -0.000000000000000000, -0.000000000000000000 ) ) ;
#15033=VECTOR ( 'NONE', #8075, 1000.000000000000000 ) ;
#15052=CIRCLE ( 'NONE', #13798, 2.000000000000000000 ) ;
#15062=ORIENTED_EDGE ( 'NONE', *, *, #9844, .T. ) ;
#15063=DIRECTION ( 'NONE',  ( -1.000000000000000000, 0.000000000000000000, 0.000000000000000000 ) ) ;
#15066=ORIENTED_EDGE ( 'NONE', *, *, #1670, .F. ) ;
#15068=CIRCLE ( 'NONE', #2878, 2.000000000000000000 ) ;
#15088=LINE ( 'NONE', #1274, #9020 ) ;
#15155=VECTOR ( 'NONE', #339, 1000.000000000000000 ) ;
#15158=ORIENTED_EDGE ( 'NONE', *, *, #752, .F. ) ;
#15185=VECTOR ( 'NONE', #7940, 1000.000000000000000 ) ;
#15202=ADVANCED_FACE ( 'NONE', ( #12232 ), #5908, .F. ) ;
#15220=( GEOMETRIC_REPRESENTATION_CONTEXT ( 3 ) GLOBAL_UNCERTAINTY_ASSIGNED_CONTEXT ( ( #7939 ) ) GLOBAL_UNIT_ASSIGNED_CONTEXT ( ( #13431, #4216, #11957 ) ) REPRESENTATION_CONTEXT ( 'NONE', 'WORKASPACE' ) );
#15224=CARTESIAN_POINT ( 'NONE',  ( 18.00000000000000355, -20.00000000000000000, -20.00000000000000000 ) ) ;
#15227=AXIS2_PLACEMENT_3D ( 'NONE', #13321, #16282, #19340 ) ;
#15236=EDGE_LOOP ( 'NONE', ( #16737, #7433, #15691 ) ) ;
#15237=AXIS2_PLACEMENT_3D ( 'NONE', #6029, #6118, #14937 ) ;
#15238=ORIENTED_EDGE ( 'NONE', *, *, #3944, .F. ) ;
#15240=VECTOR ( 'NONE', #11828, 1000.000000000000000 ) ;
#15272=ORIENTED_EDGE ( 'NONE', *, *, #6994, .F. ) ;
#15274=CYLINDRICAL_SURFACE ( 'NONE', #3630, 2.000000000000001776 ) ;
#15325=LINE ( 'NONE', #3271, #13669 ) ;
#15335=CARTESIAN_POINT ( 'NONE',  ( 75.00000000000001421, -39.99999999999998579, -20.00000000000000000 ) ) ;
#15342=LINE ( 'NONE', #6508, #8433 ) ;
#15348=DIRECTION ( 'NONE',  ( 0.000000000000000000, -1.000000000000000000, 8.673617379884035472E-16 ) ) ;
#15363=ORIENTED_EDGE ( 'NONE', *, *, #2084, .T. ) ;
#15404=EDGE_CURVE ( 'NONE', #2682, #10823, #2484, .T. ) ;
#15429=ADVANCED_FACE ( 'NONE', ( #14371 ), #955, .F. ) ;
#15441=ADVANCED_FACE ( 'NONE', ( #11623 ), #17432, .T. ) ;
#15463=FACE_OUTER_BOUND ( 'NONE', #17345, .T. ) ;
#15466=ORIENTED_EDGE ( 'NONE', *, *, #3522, .T. ) ;
#15467=DIRECTION ( 'NONE',  ( -1.000000000000000000, 0.000000000000000000, -0.000000000000000000 ) ) ;
#15470=DIRECTION ( 'NONE',  ( 3.469446951953615175E-16, -1.000000000000000000, 0.000000000000000000 ) ) ;
#15490=DIRECTION ( 'NONE',  ( 0.000000000000000000, 0.000000000000000000, 1.000000000000000000 ) ) ;
#15513=AXIS2_PLACEMENT_3D ( 'NONE', #6740, #2261, #12726 ) ;
#15526=DIRECTION ( 'NONE',  ( 1.000000000000000000, -0.000000000000000000, -0.000000000000000000 ) ) ;
#15529=STYLED_ITEM('',(#19447),#1938);
#15544=PLANE ( 'NONE',  #3842 ) ;
#15578=ORIENTED_EDGE ( 'NONE', *, *, #4024, .T. ) ;
#15585=ORIENTED_EDGE ( 'NONE', *, *, #2455, .F. ) ;
#15592=CYLINDRICAL_SURFACE ( 'NONE', #4226, 1.999999999999998224 ) ;
#15609=CARTESIAN_POINT ( 'NONE',  ( -20.00000000000000000, -19.99999999999999289, -12.00000000000000000 ) ) ;
#15619=DIRECTION ( 'NONE',  ( 1.000000000000000000, -0.000000000000000000, -0.000000000000000000 ) ) ;
#15631=VERTEX_POINT ( 'NONE', #12485 ) ;
#15633=EDGE_CURVE ( 'NONE', #17671, #5344, #4770, .T. ) ;
#15683=ORIENTED_EDGE ( 'NONE', *, *, #19251, .T. ) ;
#15687=VECTOR ( 'NONE', #9424, 1000.000000000000000 ) ;
#15691=ORIENTED_EDGE ( 'NONE', *, *, #18929, .T. ) ;
#15718=LINE ( 'NONE', #5121, #2339 ) ;
#15735=DIRECTION ( 'NONE',  ( 0.000000000000000000, 8.673617379884036458E-16, 1.000000000000000000 ) ) ;
#15751=EDGE_CURVE ( 'NONE', #2682, #9345, #15342, .T. ) ;
#15761=ORIENTED_EDGE ( 'NONE', *, *, #13409, .F. ) ;
#15773=FACE_OUTER_BOUND ( 'NONE', #98, .T. ) ;
#15775=CARTESIAN_POINT ( 'NONE',  ( -44.99999999999997158, -40.00000000000000000, -10.00000000000000000 ) ) ;
#15782=CIRCLE ( 'NONE', #6086, 2.000000000000001776 ) ;
#15792=VECTOR ( 'NONE', #18563, 1000.000000000000000 ) ;
#15817=VECTOR ( 'NONE', #3930, 1000.000000000000000 ) ;
#15823=LINE ( 'NONE', #9534, #17895 ) ;
#15838=DIRECTION ( 'NONE',  ( -0.000000000000000000, 1.000000000000000000, -0.000000000000000000 ) ) ;
#15847=EDGE_CURVE ( 'NONE', #1920, #14655, #4048, .T. ) ;
#15857=VERTEX_POINT ( 'NONE', #8174 ) ;
#15863=ORIENTED_EDGE ( 'NONE', *, *, #17794, .F. ) ;
#15866=ADVANCED_FACE ( 'NONE', ( #14245 ), #12588, .F. ) ;
#15869=DIRECTION ( 'NONE',  ( -0.000000000000000000, -0.000000000000000000, -1.000000000000000000 ) ) ;
#15872=EDGE_CURVE ( 'NONE', #14264, #17671, #18889, .T. ) ;
#15873=VERTEX_POINT ( 'NONE', #12973 ) ;
#15877=LINE ( 'NONE', #8412, #19363 ) ;
#15895=AXIS2_PLACEMENT_3D ( 'NONE', #18511, #942, #8086 ) ;
#15901=AXIS2_PLACEMENT_3D ( 'NONE', #13549, #11872, #122 ) ;
#15907=DIRECTION ( 'NONE',  ( -1.000000000000000000, 0.000000000000000000, 0.000000000000000000 ) ) ;
#15910=DIRECTION ( 'NONE',  ( 0.000000000000000000, -0.000000000000000000, 1.000000000000000000 ) ) ;
#15940=CARTESIAN_POINT ( 'NONE',  ( 75.00000000000002842, 3.000000000000000888, -5.999999999999998224 ) ) ;
#15968=CYLINDRICAL_SURFACE ( 'NONE', #13618, 1.999999999999998224 ) ;
#15972=VERTEX_POINT ( 'NONE', #4551 ) ;
#15978=VERTEX_POINT ( 'NONE', #10127 ) ;
#15986=VECTOR ( 'NONE', #10278, 1000.000000000000000 ) ;
#15998=ADVANCED_FACE ( 'NONE', ( #11788 ), #8757, .T. ) ;
#16000=CARTESIAN_POINT ( 'NONE',  ( -74.99999999999997158, -1.000000000000000000, 6.000000000000001776 ) ) ;
#16012=FACE_OUTER_BOUND ( 'NONE', #17215, .T. ) ;
#16017=PLANE ( 'NONE',  #3082 ) ;
#16035=EDGE_CURVE ( 'NONE', #13101, #514, #17699, .T. ) ;
#16036=DIRECTION ( 'NONE',  ( -0.000000000000000000, -0.000000000000000000, 1.000000000000000000 ) ) ;
#16050=EDGE_LOOP ( 'NONE', ( #4181, #1508, #7606, #10728 ) ) ;
#16061=EDGE_CURVE ( 'NONE', #9398, #965, #7192, .T. ) ;
#16062=DIRECTION ( 'NONE',  ( -3.469446951953614682E-16, 1.000000000000000000, 0.000000000000000000 ) ) ;
#16070=CARTESIAN_POINT ( 'NONE',  ( -20.00000000000000000, -19.99999999999999289, -20.00000000000000000 ) ) ;
#16073=CARTESIAN_POINT ( 'NONE',  ( 30.00000000000000000, -3.000000000000002665, -5.999999999999998224 ) ) ;
#16076=ORIENTED_EDGE ( 'NONE', *, *, #1782, .F. ) ;
#16096=FILL_AREA_STYLE ('',( #14809 ) ) ;
#16104=VECTOR ( 'NONE', #15619, 1000.000000000000000 ) ;
#16107=CARTESIAN_POINT ( 'NONE',  ( 2.449293598294706513E-15, -20.00000000000000000, -20.00000000000000000 ) ) ;
#16122=EDGE_CURVE ( 'NONE', #13131, #1122, #5021, .T. ) ;
#16125=ORIENTED_EDGE ( 'NONE', *, *, #3537, .T. ) ;
#16129=EDGE_CURVE ( 'NONE', #6347, #8396, #16513, .T. ) ;
#16131=AXIS2_PLACEMENT_3D ( 'NONE', #3352, #15490, #3258 ) ;
#16133=DIRECTION ( 'NONE',  ( 0.000000000000000000, 0.000000000000000000, 1.000000000000000000 ) ) ;
#16147=ORIENTED_EDGE ( 'NONE', *, *, #10319, .F. ) ;
#16150=EDGE_LOOP ( 'NONE', ( #14398, #4281, #5045, #16153 ) ) ;
#16153=ORIENTED_EDGE ( 'NONE', *, *, #10456, .T. ) ;
#16157=CARTESIAN_POINT ( 'NONE',  ( -72.99999999999997158, 2.999999999999999112, -5.999999999999998224 ) ) ;
#16158=VERTEX_POINT ( 'NONE', #18190 ) ;
#16160=ORIENTED_EDGE ( 'NONE', *, *, #18778, .T. ) ;
#16173=CARTESIAN_POINT ( 'NONE',  ( 0.000000000000000000, 0.000000000000000000, -10.00000000000000000 ) ) ;
#16191=DIRECTION ( 'NONE',  ( 1.000000000000000000, 0.000000000000000000, 0.000000000000000000 ) ) ;
#16212=CARTESIAN_POINT ( 'NONE',  ( 50.00000000000000000, 15.00000000000000000, 0.000000000000000000 ) ) ;
#16216=FACE_OUTER_BOUND ( 'NONE', #12101, .T. ) ;
#16269=FACE_BOUND ( 'NONE', #11314, .T. ) ;
#16273=VERTEX_POINT ( 'NONE', #2187 ) ;
#16279=ORIENTED_EDGE ( 'NONE', *, *, #3415, .F. ) ;
#16282=DIRECTION ( 'NONE',  ( 0.000000000000000000, 0.000000000000000000, -1.000000000000000000 ) ) ;
#16304=DIRECTION ( 'NONE',  ( 1.000000000000000000, 0.000000000000000000, 0.000000000000000000 ) ) ;
#16310=LINE ( 'NONE', #2884, #4312 ) ;
#16317=AXIS2_PLACEMENT_3D ( 'NONE', #10978, #5189, #3541 ) ;
#16327=FACE_OUTER_BOUND ( 'NONE', #19141, .T. ) ;
#16343=ORIENTED_EDGE ( 'NONE', *, *, #1539, .T. ) ;
#16349=EDGE_CURVE ( 'NONE', #14264, #15631, #3945, .T. ) ;
#16369=EDGE_LOOP ( 'NONE', ( #12387, #8170, #17747, #8175 ) ) ;
#16378=VECTOR ( 'NONE', #7103, 1000.000000000000000 ) ;
#16392=CARTESIAN_POINT ( 'NONE',  ( 18.00000000000000355, -20.00000000000000000, -12.00000000000000000 ) ) ;
#16399=VERTEX_POINT ( 'NONE', #10109 ) ;
#16433=VECTOR ( 'NONE', #5194, 1000.000000000000000 ) ;
#16447=ORIENTED_EDGE ( 'NONE', *, *, #11542, .T. ) ;
#16460=VECTOR ( 'NONE', #18229, 1000.000000000000000 ) ;
#16461=CARTESIAN_POINT ( 'NONE',  ( 2.449293598294706513E-15, -20.00000000000000000, -20.00000000000000000 ) ) ;
#16463=ORIENTED_EDGE ( 'NONE', *, *, #4827, .T. ) ;
#16471=EDGE_CURVE ( 'NONE', #15972, #13265, #6257, .T. ) ;
#16475=PLANE ( 'NONE',  #5670 ) ;
#16513=LINE ( 'NONE', #18088, #10 ) ;
#16515=ORIENTED_EDGE ( 'NONE', *, *, #16471, .F. ) ;
#16536=ORIENTED_EDGE ( 'NONE', *, *, #4224, .F. ) ;
#16542=CARTESIAN_POINT ( 'NONE',  ( -74.99999999999997158, 1.000000000000000000, 6.000000000000000000 ) ) ;
#16574=DIRECTION ( 'NONE',  ( -1.000000000000000000, 0.000000000000000000, 0.000000000000000000 ) ) ;
#16612=EDGE_CURVE ( 'NONE', #6443, #6347, #3446, .T. ) ;
#16615=VECTOR ( 'NONE', #12751, 1000.000000000000000 ) ;
#16685=FACE_OUTER_BOUND ( 'NONE', #2944, .T. ) ;
#16700=ADVANCED_FACE ( 'NONE', ( #3165 ), #16883, .F. ) ;
#16711=CARTESIAN_POINT ( 'NONE',  ( 30.00000000000000000, -40.00000000000000000, -5.999999999999998224 ) ) ;
#16723=CARTESIAN_POINT ( 'NONE',  ( 50.00000000000000000, 15.00000000000000000, -4.000000000000003553 ) ) ;
#16726=ORIENTED_EDGE ( 'NONE', *, *, #11781, .F. ) ;
#16737=ORIENTED_EDGE ( 'NONE', *, *, #3110, .F. ) ;
#16744=LINE ( 'NONE', #3311, #11182 ) ;
#16750=VERTEX_POINT ( 'NONE', #14199 ) ;
#16751=ORIENTED_EDGE ( 'NONE', *, *, #10519, .F. ) ;
#16761=EDGE_CURVE ( 'NONE', #12225, #14264, #18558, .T. ) ;
#16810=CARTESIAN_POINT ( 'NONE',  ( -74.99999999999997158, -39.99999999999998579, 10.00000000000000000 ) ) ;
#16825=ORIENTED_EDGE ( 'NONE', *, *, #19251, .F. ) ;
#16836=EDGE_CURVE ( 'NONE', #590, #1122, #17243, .T. ) ;
#16840=CONICAL_SURFACE ( 'NONE', #8363, 4.000000000000003553, 1.029744260000001077 ) ;
#16843=EDGE_CURVE ( 'NONE', #15857, #16855, #14404, .T. ) ;
#16855=VERTEX_POINT ( 'NONE', #784 ) ;
#16863=PLANE ( 'NONE',  #662 ) ;
#16868=LINE ( 'NONE', #3245, #4888 ) ;
#16873=CARTESIAN_POINT ( 'NONE',  ( 32.00000000000000000, -3.000000000000000000, -5.999999999999998224 ) ) ;
#16883=PLANE ( 'NONE',  #14714 ) ;
#16885=EDGE_CURVE ( 'NONE', #3214, #16273, #6568, .T. ) ;
#16889=DIRECTION ( 'NONE',  ( 0.000000000000000000, 0.000000000000000000, -1.000000000000000000 ) ) ;
#16891=LINE ( 'NONE', #3454, #11579 ) ;
#16907=EDGE_LOOP ( 'NONE', ( #9347, #2899, #13515, #14057 ) ) ;
#16925=ORIENTED_EDGE ( 'NONE', *, *, #265, .T. ) ;
#16958=ADVANCED_FACE ( 'NONE', ( #13585 ), #7513, .F. ) ;
#16959=EDGE_LOOP ( 'NONE', ( #14930, #6235, #13582, #2749 ) ) ;
#16965=DIRECTION ( 'NONE',  ( -0.000000000000000000, -0.000000000000000000, 1.000000000000000000 ) ) ;
#16970=CIRCLE ( 'NONE', #8502, 2.000000000000000000 ) ;
#16982=ORIENTED_EDGE ( 'NONE', *, *, #7250, .T. ) ;
#16989=DIRECTION ( 'NONE',  ( -0.000000000000000000, -0.000000000000000000, 1.000000000000000000 ) ) ;
#16999=ORIENTED_EDGE ( 'NONE', *, *, #10319, .T. ) ;
#17016=EDGE_CURVE ( 'NONE', #2111, #16399, #1784, .T. ) ;
#17018=LINE ( 'NONE', #16723, #5041 ) ;
#17028=VERTEX_POINT ( 'NONE', #9025 ) ;
#17047=ORIENTED_EDGE ( 'NONE', *, *, #3110, .T. ) ;
#17058=PRODUCT_DEFINITION ( 'UNKNOWN', '', #14167, #11049 ) ;
#17067=CARTESIAN_POINT ( 'NONE',  ( -30.00000000000000000, -40.00000000000000000, 12.50000000000000000 ) ) ;
#17105=VECTOR ( 'NONE', #2941, 1000.000000000000000 ) ;
#17118=EDGE_CURVE ( 'NONE', #11964, #15631, #694, .T. ) ;
#17120=ORIENTED_EDGE ( 'NONE', *, *, #2455, .T. ) ;
#17127=LINE ( 'NONE', #2229, #4473 ) ;
#17152=DIRECTION ( 'NONE',  ( -1.000000000000000000, 0.000000000000000000, 0.000000000000000000 ) ) ;
#17159=LINE ( 'NONE', #11546, #4023 ) ;
#17169=FACE_OUTER_BOUND ( 'NONE', #5672, .T. ) ;
#17181=ADVANCED_FACE ( 'NONE', ( #17169 ), #4418, .F. ) ;
#17196=AXIS2_PLACEMENT_3D ( 'NONE', #18911, #17427, #11332 ) ;
#17215=EDGE_LOOP ( 'NONE', ( #6559, #1528, #6326, #7516 ) ) ;
#17239=DIRECTION ( 'NONE',  ( -0.000000000000000000, -0.000000000000000000, -1.000000000000000000 ) ) ;
#17243=CIRCLE ( 'NONE', #11576, 2.000000000000001776 ) ;
#17246=AXIS2_PLACEMENT_3D ( 'NONE', #14800, #3150, #4616 ) ;
#17252=AXIS2_PLACEMENT_3D ( 'NONE', #2790, #2698, #13458 ) ;
#17268=ORIENTED_EDGE ( 'NONE', *, *, #17016, .T. ) ;
#17284=APPLICATION_CONTEXT ( 'automotive_design' ) ;
#17290=CIRCLE ( 'NONE', #2265, 1.999999999999998224 ) ;
#17295=EDGE_LOOP ( 'NONE', ( #10925, #13032, #3036, #6617 ) ) ;
#17306=DIRECTION ( 'NONE',  ( -1.000000000000000000, 0.000000000000000000, 0.000000000000000000 ) ) ;
#17319=LINE ( 'NONE', #3971, #6182 ) ;
#17345=EDGE_LOOP ( 'NONE', ( #3237, #11177, #1172, #3875 ) ) ;
#17352=DIRECTION ( 'NONE',  ( 0.000000000000000000, 0.000000000000000000, -1.000000000000000000 ) ) ;
#17355=CONICAL_SURFACE ( 'NONE', #1070, 4.000000000000003553, 1.029744260000001077 ) ;
#17372=CARTESIAN_POINT ( 'NONE',  ( 2.449293598294706513E-15, -20.00000000000000000, -20.00000000000000000 ) ) ;
#17387=CARTESIAN_POINT ( 'NONE',  ( -74.99999999999998579, -7.500000000000027534, -10.00000000000000000 ) ) ;
#17391=LINE ( 'NONE', #5783, #3657 ) ;
#17407=DIRECTION ( 'NONE',  ( 0.000000000000000000, 1.000000000000000000, 0.000000000000000000 ) ) ;
#17427=DIRECTION ( 'NONE',  ( 0.000000000000000000, 0.000000000000000000, -1.000000000000000000 ) ) ;
#17432=CYLINDRICAL_SURFACE ( 'NONE', #18768, 2.000000000000001776 ) ;
#17440=EDGE_LOOP ( 'NONE', ( #6283, #13358, #1710, #8393 ) ) ;
#17452=ORIENTED_EDGE ( 'NONE', *, *, #10519, .T. ) ;
#17457=EDGE_CURVE ( 'NONE', #11891, #5733, #13034, .T. ) ;
#17478=CARTESIAN_POINT ( 'NONE',  ( -44.99999999999997158, -7.499999999999971578, -20.00000000000000000 ) ) ;
#17499=CARTESIAN_POINT ( 'NONE',  ( -20.00000000000000000, -19.99999999999999289, -20.00000000000000000 ) ) ;
#17506=ORIENTED_EDGE ( 'NONE', *, *, #8931, .F. ) ;
#17524=ORIENTED_EDGE ( 'NONE', *, *, #18992, .F. ) ;
#17526=ORIENTED_EDGE ( 'NONE', *, *, #15847, .F. ) ;
#17563=VECTOR ( 'NONE', #2306, 1000.000000000000000 ) ;
#17585=ORIENTED_EDGE ( 'NONE', *, *, #12167, .T. ) ;
#17586=VECTOR ( 'NONE', #17955, 1000.000000000000000 ) ;
#17607=DIRECTION ( 'NONE',  ( 0.000000000000000000, 0.000000000000000000, -1.000000000000000000 ) ) ;
#17608=ORIENTED_EDGE ( 'NONE', *, *, #16471, .T. ) ;
#17618=EDGE_CURVE ( 'NONE', #14876, #2713, #5985, .T. ) ;
#17623=CARTESIAN_POINT ( 'NONE',  ( 73.00000000000002842, -1.000000000000000000, 6.000000000000001776 ) ) ;
#17628=ORIENTED_EDGE ( 'NONE', *, *, #12425, .F. ) ;
#17651=ORIENTED_EDGE ( 'NONE', *, *, #19014, .F. ) ;
#17656=ADVANCED_FACE ( 'NONE', ( #7445 ), #16475, .F. ) ;
#17667=EDGE_CURVE ( 'NONE', #6445, #9743, #10040, .T. ) ;
#17671=VERTEX_POINT ( 'NONE', #8301 ) ;
#17673=ADVANCED_FACE ( 'NONE', ( #7917 ), #16863, .F. ) ;
#17687=DIRECTION ( 'NONE',  ( -1.000000000000000000, 0.000000000000000000, 0.000000000000000000 ) ) ;
#17695=CARTESIAN_POINT ( 'NONE',  ( 32.00000000000000000, -1.000000000000000000, 6.000000000000001776 ) ) ;
#17699=LINE ( 'NONE', #1511, #13440 ) ;
#17710=FACE_OUTER_BOUND ( 'NONE', #9177, .T. ) ;
#17740=EDGE_LOOP ( 'NONE', ( #16125, #10801, #3382, #685, #5844, #14166, #17989, #18310 ) ) ;
#17747=ORIENTED_EDGE ( 'NONE', *, *, #3643, .T. ) ;
#17764=LINE ( 'NONE', #2962, #3085 ) ;
#17779=CARTESIAN_POINT ( 'NONE',  ( -65.14999999999996305, 32.50000000000001421, 10.00000000000000000 ) ) ;
#17794=EDGE_CURVE ( 'NONE', #10823, #2682, #1245, .T. ) ;
#17840=VERTEX_POINT ( 'NONE', #8153 ) ;
#17849=CIRCLE ( 'NONE', #9364, 2.649999999999985700 ) ;
#17850=ORIENTED_EDGE ( 'NONE', *, *, #10811, .F. ) ;
#17854=DIRECTION ( 'NONE',  ( 0.000000000000000000, 0.000000000000000000, 1.000000000000000000 ) ) ;
#17865=DIRECTION ( 'NONE',  ( -0.8571673013836855759, 0.000000000000000000, -0.5150380737757258576 ) ) ;
#17867=DIRECTION ( 'NONE',  ( 0.000000000000000000, 0.000000000000000000, 1.000000000000000000 ) ) ;
#17880=DIRECTION ( 'NONE',  ( 1.000000000000000000, -0.000000000000000000, -0.000000000000000000 ) ) ;
#17895=VECTOR ( 'NONE', #15526, 1000.000000000000000 ) ;
#17899=EDGE_CURVE ( 'NONE', #1343, #8396, #14128, .T. ) ;
#17911=AXIS2_PLACEMENT_3D ( 'NONE', #3177, #11980, #220 ) ;
#17914=VERTEX_POINT ( 'NONE', #10998 ) ;
#17955=DIRECTION ( 'NONE',  ( 0.000000000000000000, -1.000000000000000000, 0.000000000000000000 ) ) ;
#17970=SURFACE_SIDE_STYLE ('',( #4529 ) ) ;
#17973=ORIENTED_EDGE ( 'NONE', *, *, #18992, .T. ) ;
#17975=ADVANCED_FACE ( 'NONE', ( #16012 ), #10298, .F. ) ;
#17989=ORIENTED_EDGE ( 'NONE', *, *, #7250, .F. ) ;
#17999=LINE ( 'NONE', #8956, #7639 ) ;
#18005=AXIS2_PLACEMENT_3D ( 'NONE', #17372, #6960, #14405 ) ;
#18017=FACE_OUTER_BOUND ( 'NONE', #14963, .T. ) ;
#18032=ORIENTED_EDGE ( 'NONE', *, *, #50, .F. ) ;
#18036=EDGE_CURVE ( 'NONE', #10379, #13579, #10009, .T. ) ;
#18056=ADVANCED_FACE ( 'NONE', ( #8739 ), #10196, .F. ) ;
#18088=CARTESIAN_POINT ( 'NONE',  ( 75.00000000000001421, -7.499999999999971578, -10.00000000000000000 ) ) ;
#18102=EDGE_CURVE ( 'NONE', #16158, #15972, #5699, .T. ) ;
#18109=ORIENTED_EDGE ( 'NONE', *, *, #5919, .F. ) ;
#18141=CARTESIAN_POINT ( 'NONE',  ( 22.00000000000000000, -20.00000000000000000, -20.00000000000000000 ) ) ;
#18146=AXIS2_PLACEMENT_3D ( 'NONE', #1663, #18523, #5066 ) ;
#18151=CARTESIAN_POINT ( 'NONE',  ( 75.00000000000002842, -39.99999999999998579, 10.00000000000000000 ) ) ;
#18152=CARTESIAN_POINT ( 'NONE',  ( -18.00000000000000355, -19.99999999999999289, -20.00000000000000000 ) ) ;
#18190=CARTESIAN_POINT ( 'NONE',  ( 20.00000000000000000, -20.00000000000000000, -10.79827876554711530 ) ) ;
#18207=AXIS2_PLACEMENT_3D ( 'NONE', #16461, #7526, #10549 ) ;
#18224=EDGE_LOOP ( 'NONE', ( #11201, #528, #16279, #12042, #3040 ) ) ;
#18229=DIRECTION ( 'NONE',  ( 0.000000000000000000, 0.000000000000000000, -1.000000000000000000 ) ) ;
#18266=LINE ( 'NONE', #1979, #15185 ) ;
#18279=ORIENTED_EDGE ( 'NONE', *, *, #17457, .F. ) ;
#18285=DIRECTION ( 'NONE',  ( 0.000000000000000000, -1.000000000000000000, 0.000000000000000000 ) ) ;
#18310=ORIENTED_EDGE ( 'NONE', *, *, #11541, .T. ) ;
#18317=CARTESIAN_POINT ( 'NONE',  ( -72.99999999999997158, 1.000000000000000000, -5.999999999999998224 ) ) ;
#18320=CARTESIAN_POINT ( 'NONE',  ( -20.00000000000000000, -19.99999999999999289, -10.79827876554711530 ) ) ;
#18327=FACE_BOUND ( 'NONE', #14985, .T. ) ;
#18354=CARTESIAN_POINT ( 'NONE',  ( 73.00000000000000000, 1.000000000000000000, 6.000000000000000000 ) ) ;
#18362=CARTESIAN_POINT ( 'NONE',  ( -74.99999999999997158, -39.99999999999998579, 10.00000000000000000 ) ) ;
#18373=DIRECTION ( 'NONE',  ( -1.000000000000000000, 9.251858538542972814E-17, -0.000000000000000000 ) ) ;
#18380=CARTESIAN_POINT ( 'NONE',  ( -44.99999999999997158, -7.499999999999971578, -10.00000000000000000 ) ) ;
#18407=ORIENTED_EDGE ( 'NONE', *, *, #12147, .T. ) ;
#18437=FACE_BOUND ( 'NONE', #16907, .T. ) ;
#18446=PLANE ( 'NONE',  #3392 ) ;
#18451=AXIS2_PLACEMENT_3D ( 'NONE', #6928, #18914, #11429 ) ;
#18461=DIRECTION ( 'NONE',  ( 0.000000000000000000, 8.673617379884036458E-16, 1.000000000000000000 ) ) ;
#18467=VECTOR ( 'NONE', #13384, 1000.000000000000000 ) ;
#18485=VECTOR ( 'NONE', #17865, 1000.000000000000114 ) ;
#18500=ORIENTED_EDGE ( 'NONE', *, *, #7036, .T. ) ;
#18501=LINE ( 'NONE', #3389, #15033 ) ;
#18511=CARTESIAN_POINT ( 'NONE',  ( 32.00000000000000000, 3.000000000000000000, 5.999999999999998224 ) ) ;
#18522=ORIENTED_EDGE ( 'NONE', *, *, #8208, .T. ) ;
#18523=DIRECTION ( 'NONE',  ( 0.000000000000000000, 0.000000000000000000, 1.000000000000000000 ) ) ;
#18533=LINE ( 'NONE', #5074, #12080 ) ;
#18540=CARTESIAN_POINT ( 'NONE',  ( -44.99999999999997158, -40.00000000000000000, -10.00000000000000000 ) ) ;
#18544=EDGE_CURVE ( 'NONE', #16273, #5461, #1432, .T. ) ;
#18552=VERTEX_POINT ( 'NONE', #4667 ) ;
#18553=DIRECTION ( 'NONE',  ( 1.000000000000000000, -0.000000000000000000, 0.000000000000000000 ) ) ;
#18556=EDGE_LOOP ( 'NONE', ( #7786, #12440, #9950, #5684 ) ) ;
#18558=LINE ( 'NONE', #12642, #9078 ) ;
#18563=DIRECTION ( 'NONE',  ( -0.000000000000000000, -0.000000000000000000, 1.000000000000000000 ) ) ;
#18581=ORIENTED_EDGE ( 'NONE', *, *, #15751, .F. ) ;
#18598=CARTESIAN_POINT ( 'NONE',  ( -74.99999999999997158, -39.99999999999998579, 10.00000000000000000 ) ) ;
#18633=FACE_OUTER_BOUND ( 'NONE', #10607, .T. ) ;
#18639=ORIENTED_EDGE ( 'NONE', *, *, #17794, .T. ) ;
#18655=CARTESIAN_POINT ( 'NONE',  ( -29.99999999999999645, -39.99999999999998579, -12.49999999999999822 ) ) ;
#18670=CONICAL_SURFACE ( 'NONE', #9881, 1.999999999999998224, 1.029744259999999745 ) ;
#18739=VECTOR ( 'NONE', #3373, 1000.000000000000000 ) ;
#18766=ORIENTED_EDGE ( 'NONE', *, *, #12623, .T. ) ;
#18768=AXIS2_PLACEMENT_3D ( 'NONE', #2821, #8784, #7509 ) ;
#18778=EDGE_CURVE ( 'NONE', #16273, #3214, #2838, .T. ) ;
#18790=ORIENTED_EDGE ( 'NONE', *, *, #16035, .T. ) ;
#18814=ADVANCED_FACE ( 'NONE', ( #18975 ), #725, .F. ) ;
#18840=VECTOR ( 'NONE', #7884, 1000.000000000000000 ) ;
#18841=FACE_OUTER_BOUND ( 'NONE', #16369, .T. ) ;
#18843=MECHANICAL_DESIGN_GEOMETRIC_PRESENTATION_REPRESENTATION('',(#1921),#6297);
#18868=DIRECTION ( 'NONE',  ( -1.000000000000000000, -3.469446951953615175E-16, -0.000000000000000000 ) ) ;
#18887=EDGE_CURVE ( 'NONE', #11691, #3485, #3863, .T. ) ;
#18889=LINE ( 'NONE', #5424, #7485 ) ;
#18894=ORIENTED_EDGE ( 'NONE', *, *, #11171, .F. ) ;
#18911=CARTESIAN_POINT ( 'NONE',  ( 0.000000000000000000, 0.000000000000000000, -10.00000000000000000 ) ) ;
#18914=DIRECTION ( 'NONE',  ( -0.000000000000000000, -0.000000000000000000, 1.000000000000000000 ) ) ;
#18924=LINE ( 'NONE', #15775, #11098 ) ;
#18929=EDGE_CURVE ( 'NONE', #7086, #928, #335, .T. ) ;
#18944=PLANE ( 'NONE',  #13617 ) ;
#18962=AXIS2_PLACEMENT_3D ( 'NONE', #12009, #2820, #4674 ) ;
#18975=FACE_OUTER_BOUND ( 'NONE', #1922, .T. ) ;
#18992=EDGE_CURVE ( 'NONE', #4430, #1140, #5026, .T. ) ;
#19014=EDGE_CURVE ( 'NONE', #11065, #13816, #13488, .T. ) ;
#19031=CARTESIAN_POINT ( 'NONE',  ( -62.49999999999997158, 32.50000000000001421, 10.00000000000000000 ) ) ;
#19042=CIRCLE ( 'NONE', #10553, 2.649999999999985700 ) ;
#19046=DIRECTION ( 'NONE',  ( 0.000000000000000000, 0.000000000000000000, -1.000000000000000000 ) ) ;
#19054=( NAMED_UNIT ( * ) PLANE_ANGLE_UNIT ( ) SI_UNIT ( $, .RADIAN. ) );
#19055=ADVANCED_FACE ( 'NONE', ( #13556, #11687 ), #14828, .T. ) ;
#19083=CARTESIAN_POINT ( 'NONE',  ( -72.99999999999997158, -3.000000000000000000, -20.00000000000000000 ) ) ;
#19084=ORIENTED_EDGE ( 'NONE', *, *, #8199, .F. ) ;
#19106=DIRECTION ( 'NONE',  ( 0.000000000000000000, -1.000000000000000000, -0.000000000000000000 ) ) ;
#19141=EDGE_LOOP ( 'NONE', ( #13525, #8478, #1058, #2412 ) ) ;
#19147=CARTESIAN_POINT ( 'NONE',  ( 22.00000000000000000, -20.00000000000000000, -12.00000000000000000 ) ) ;
#19161=PRESENTATION_STYLE_ASSIGNMENT (( #4432 ) ) ;
#19166=DIRECTION ( 'NONE',  ( -1.000000000000000000, 0.000000000000000000, 0.000000000000000000 ) ) ;
#19182=DIRECTION ( 'NONE',  ( 0.000000000000000000, 0.000000000000000000, 1.000000000000000000 ) ) ;
#19206=VERTEX_POINT ( 'NONE', #3460 ) ;
#19222=LINE ( 'NONE', #1259, #15240 ) ;
#19230=DIRECTION ( 'NONE',  ( -0.000000000000000000, 0.000000000000000000, -1.000000000000000000 ) ) ;
#19236=EDGE_CURVE ( 'NONE', #13816, #16855, #7766, .T. ) ;
#19243=VECTOR ( 'NONE', #4075, 1000.000000000000000 ) ;
#19251=EDGE_CURVE ( 'NONE', #7579, #4866, #6304, .T. ) ;
#19254=SHAPE_REPRESENTATION_RELATIONSHIP ( 'NONE' , 'NONE' ,  #6546, #9419 ) ;
#19276=CIRCLE ( 'NONE', #11395, 2.000000000000000000 ) ;
#19284=ORIENTED_EDGE ( 'NONE', *, *, #15020, .F. ) ;
#19304=CYLINDRICAL_SURFACE ( 'NONE', #7487, 2.000000000000001776 ) ;
#19306=EDGE_CURVE ( 'NONE', #9398, #11277, #12363, .T. ) ;
#19327=ORIENTED_EDGE ( 'NONE', *, *, #5259, .T. ) ;
#19333=DIRECTION ( 'NONE',  ( -0.000000000000000000, -0.000000000000000000, -1.000000000000000000 ) ) ;
#19340=DIRECTION ( 'NONE',  ( -1.000000000000000000, 0.000000000000000000, 0.000000000000000000 ) ) ;
#19363=VECTOR ( 'NONE', #7246, 1000.000000000000000 ) ;
#19365=CARTESIAN_POINT ( 'NONE',  ( 32.00000000000000000, 1.000000000000000000, -5.999999999999998224 ) ) ;
#19373=CARTESIAN_POINT ( 'NONE',  ( 75.00000000000001421, -39.99999999999998579, -20.00000000000000000 ) ) ;
#19383=DIRECTION ( 'NONE',  ( -1.000000000000000000, 0.000000000000000000, 0.000000000000000000 ) ) ;
#19413=DIRECTION ( 'NONE',  ( 0.000000000000000000, -0.000000000000000000, 1.000000000000000000 ) ) ;
#19441=COLOUR_RGB('Dark Blue',0.08,0.2,0.34);
#19442=FILL_AREA_STYLE_COLOUR('',#19441);
#19443=FILL_AREA_STYLE('',(#19442));
#19444=SURFACE_STYLE_FILL_AREA(#19443);
#19445=SURFACE_SIDE_STYLE('',(#19444));
#19446=SURFACE_STYLE_USAGE(.BOTH.,#19445);
#19447=PRESENTATION_STYLE_ASSIGNMENT((#19446));
ENDSEC;
END-ISO-10303-21;
